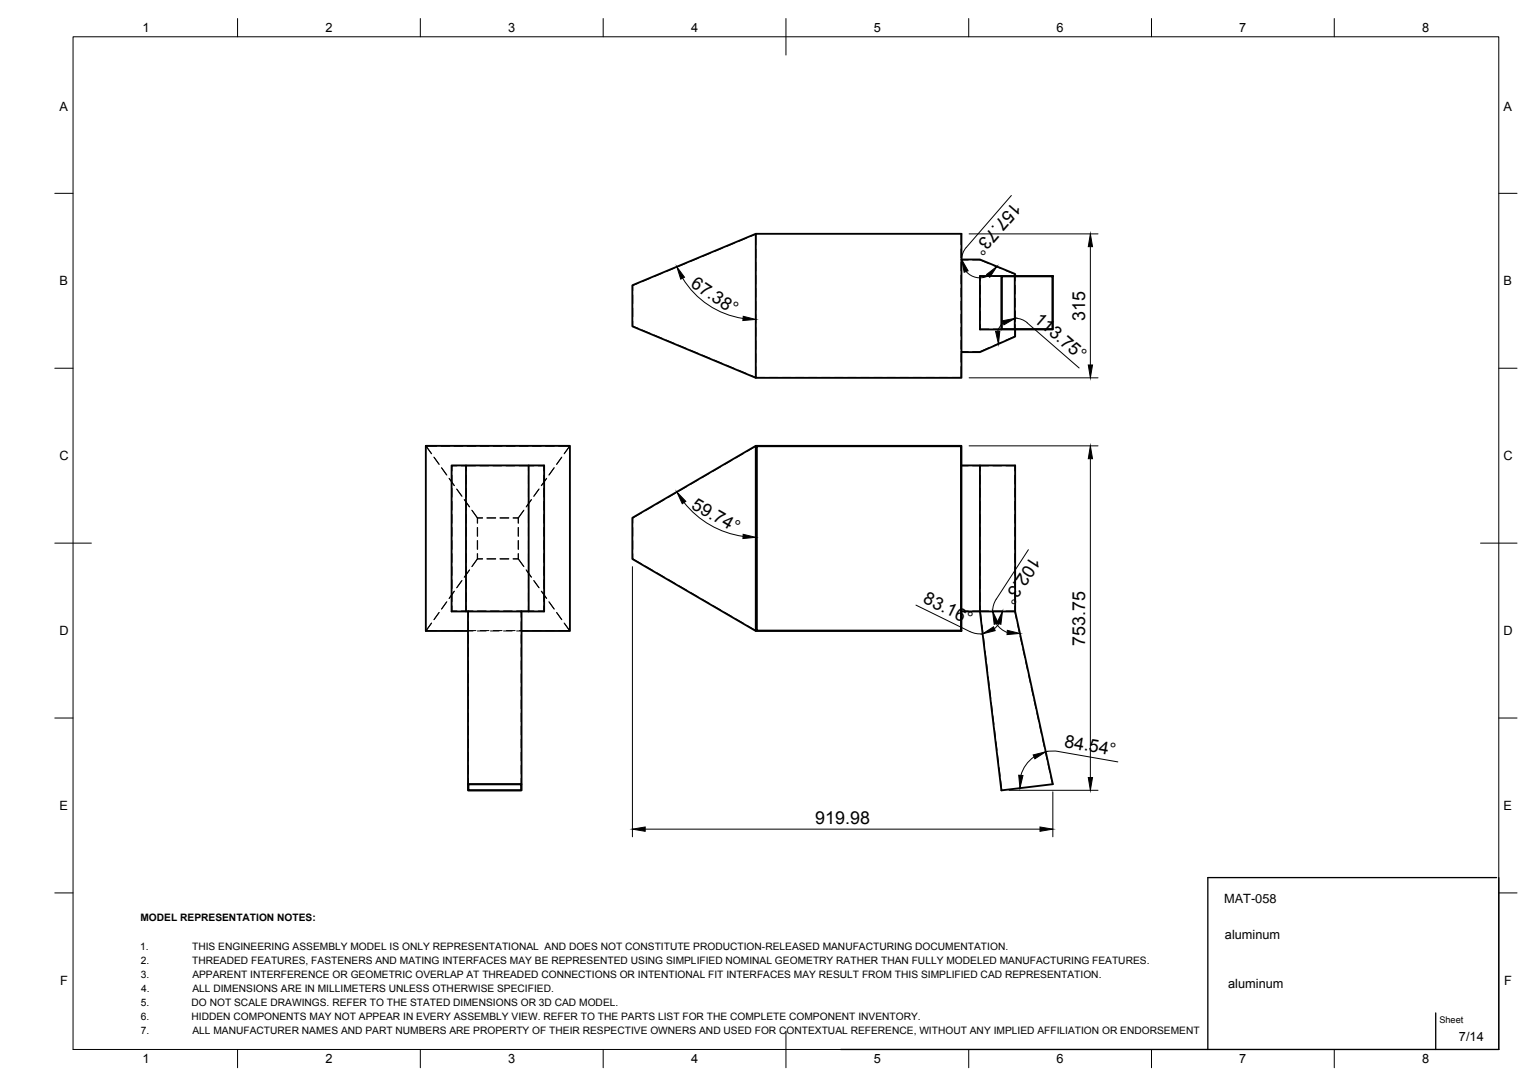
ISO-10303-21;
HEADER;
FILE_DESCRIPTION (('STEP AP214'),
    '1' );
FILE_NAME ('aluminum.step',
    '2026-10-21T17:54:40',
    ( '' ),
    ( '' ),
    'SwSTEP 2.0',
    'SolidWorks 2026',
    '' );
FILE_SCHEMA (( 'AUTOMOTIVE_DESIGN' ));
ENDSEC;

DATA;
#241=CARTESIAN_POINT ( 'NONE',  ( -208.1473046169136580, -154.8119894309599260, 472.8425600500171981 ) ) ;
#279=ORIENTED_EDGE ( 'NONE', *, *, #33326, .F. ) ;
#332=DIRECTION ( 'NONE',  ( 0.000000000000000000, -1.000000000000000000, 0.000000000000000000 ) ) ;
#357=VERTEX_POINT ( 'NONE', #3480 ) ;
#385=DIRECTION ( 'NONE',  ( 0.000000000000000000, -1.000000000000000000, 0.000000000000000000 ) ) ;
#451=CARTESIAN_POINT ( 'NONE',  ( -5.647304616913629616, 54.43801056904005975, 22.84256005001721945 ) ) ;
#457=CARTESIAN_POINT ( 'NONE',  ( 153.2026953830863647, 69.44873401059479079, -93.79675437945476801 ) ) ;
#484=DIRECTION ( 'NONE',  ( 0.1191452206184307472, 0.000000000000000000, -0.9928768384869219865 ) ) ;
#499=VECTOR ( 'NONE', #28091, 1000.000000000000000 ) ;
#615=DIRECTION ( 'NONE',  ( -0.000000000000000000, -1.000000000000000000, 0.000000000000000000 ) ) ;
#668=ORIENTED_EDGE ( 'NONE', *, *, #6729, .T. ) ;
#693=DIRECTION ( 'NONE',  ( 0.000000000000000000, -0.000000000000000000, 1.000000000000000000 ) ) ;
#702=ORIENTED_EDGE ( 'NONE', *, *, #9302, .T. ) ;
#814=CARTESIAN_POINT ( 'NONE',  ( -208.1473046169136580, -154.8119894309599260, 472.8425600500171981 ) ) ;
#959=ORIENTED_EDGE ( 'NONE', *, *, #6440, .T. ) ;
#975=CARTESIAN_POINT ( 'NONE',  ( 370.7621192902014968, 70.03596893647589638, -94.69675437945477370 ) ) ;
#987=DIRECTION ( 'NONE',  ( 1.000000000000000000, 0.000000000000000000, 0.000000000000000000 ) ) ;
#1016=VERTEX_POINT ( 'NONE', #25216 ) ;
#1060=EDGE_CURVE ( 'NONE', #41472, #40281, #17516, .T. ) ;
#1066=EDGE_CURVE ( 'NONE', #38528, #20059, #40122, .T. ) ;
#1071=ORIENTED_EDGE ( 'NONE', *, *, #6720, .F. ) ;
#1073=VECTOR ( 'NONE', #36151, 1000.000000000000114 ) ;
#1156=VECTOR ( 'NONE', #18949, 1000.000000000000000 ) ;
#1211=VERTEX_POINT ( 'NONE', #8004 ) ;
#1227=ORIENTED_EDGE ( 'NONE', *, *, #36593, .T. ) ;
#1314=VECTOR ( 'NONE', #13309, 1000.000000000000114 ) ;
#1326=ORIENTED_EDGE ( 'NONE', *, *, #18380, .F. ) ;
#1347=VECTOR ( 'NONE', #6757, 1000.000000000000114 ) ;
#1376=ADVANCED_FACE ( 'NONE', ( #40059 ), #40304, .F. ) ;
#1429=CARTESIAN_POINT ( 'NONE',  ( -556.8973046169135159, 54.43801056904003133, -64.63743994998280584 ) ) ;
#1492=LINE ( 'NONE', #20466, #38729 ) ;
#1712=DIRECTION ( 'NONE',  ( -1.000000000000000000, -0.000000000000000000, 0.000000000000000000 ) ) ;
#1716=CARTESIAN_POINT ( 'NONE',  ( 370.7621192902014968, 70.03596893647589638, -93.79675437945476801 ) ) ;
#1719=EDGE_CURVE ( 'NONE', #25392, #44652, #50206, .T. ) ;
#1752=ORIENTED_EDGE ( 'NONE', *, *, #22020, .F. ) ;
#1804=EDGE_CURVE ( 'NONE', #31856, #4890, #4338, .T. ) ;
#1839=FACE_OUTER_BOUND ( 'NONE', #12739, .T. ) ;
#1958=ORIENTED_EDGE ( 'NONE', *, *, #22698, .T. ) ;
#2000=CARTESIAN_POINT ( 'NONE',  ( -164.4973046169135955, -66.40178110878292728, -93.79675437945473959 ) ) ;
#2068=LINE ( 'NONE', #13349, #48206 ) ;
#2078=VECTOR ( 'NONE', #9444, 1000.000000000000227 ) ;
#2117=DIRECTION ( 'NONE',  ( 0.000000000000000000, -0.9253776417389547593, -0.3790464617558786942 ) ) ;
#2152=LINE ( 'NONE', #37326, #22207 ) ;
#2162=EDGE_LOOP ( 'NONE', ( #42165, #11431, #22910, #39612 ) ) ;
#2201=FACE_OUTER_BOUND ( 'NONE', #47299, .T. ) ;
#2211=ORIENTED_EDGE ( 'NONE', *, *, #2519, .F. ) ;
#2213=CARTESIAN_POINT ( 'NONE',  ( -5.647304616913629616, 160.1880105690400171, 472.8425600500173118 ) ) ;
#2225=ORIENTED_EDGE ( 'NONE', *, *, #29896, .T. ) ;
#2275=FACE_OUTER_BOUND ( 'NONE', #44624, .T. ) ;
#2284=ORIENTED_EDGE ( 'NONE', *, *, #38775, .F. ) ;
#2287=ADVANCED_FACE ( 'NONE', ( #1839 ), #41087, .T. ) ;
#2307=FACE_OUTER_BOUND ( 'NONE', #7610, .T. ) ;
#2377=PLANE ( 'NONE',  #19234 ) ;
#2481=CARTESIAN_POINT ( 'NONE',  ( 38.83576208387757589, 47.08801056904012228, 741.9425600500172777 ) ) ;
#2519=EDGE_CURVE ( 'NONE', #29402, #34186, #39530, .T. ) ;
#2583=CARTESIAN_POINT ( 'NONE',  ( -164.4973046169135955, 53.53801056904005407, -18.45589678844777382 ) ) ;
#2692=ADVANCED_FACE ( 'NONE', ( #36959 ), #36444, .T. ) ;
#2711=EDGE_LOOP ( 'NONE', ( #23565, #14957, #15394, #19348 ) ) ;
#2742=DIRECTION ( 'NONE',  ( -0.9770330068457271366, 0.000000000000000000, -0.2130880182788259247 ) ) ;
#2751=ORIENTED_EDGE ( 'NONE', *, *, #10925, .T. ) ;
#2770=AXIS2_PLACEMENT_3D ( 'NONE', #14804, #37669, #2742 ) ;
#2832=ORIENTED_EDGE ( 'NONE', *, *, #9784, .F. ) ;
#2859=ORIENTED_EDGE ( 'NONE', *, *, #15510, .T. ) ;
#2862=DIRECTION ( 'NONE',  ( 0.000000000000000000, 0.9152942571496521795, -0.4027858274925601445 ) ) ;
#2909=ORIENTED_EDGE ( 'NONE', *, *, #9784, .T. ) ;
#3005=CARTESIAN_POINT ( 'NONE',  ( 154.1026953830863420, -98.56198943095992604, -17.65743994998277699 ) ) ;
#3023=EDGE_LOOP ( 'NONE', ( #44750, #47253, #35868, #13821, #14713 ) ) ;
#3087=LINE ( 'NONE', #10042, #48814 ) ;
#3208=VECTOR ( 'NONE', #19916, 1000.000000000000000 ) ;
#3242=FACE_OUTER_BOUND ( 'NONE', #8976, .T. ) ;
#3351=DIRECTION ( 'NONE',  ( 0.000000000000000000, 0.000000000000000000, 1.000000000000000000 ) ) ;
#3374=VECTOR ( 'NONE', #29459, 1000.000000000000000 ) ;
#3480=CARTESIAN_POINT ( 'NONE',  ( -50.64730461691362962, -42.31198943095992604, 742.8425600500171413 ) ) ;
#3541=LINE ( 'NONE', #46871, #45418 ) ;
#3553=EDGE_CURVE ( 'NONE', #20088, #22621, #48242, .T. ) ;
#3577=AXIS2_PLACEMENT_3D ( 'NONE', #25346, #33059, #13534 ) ;
#3706=PLANE ( 'NONE',  #4301 ) ;
#3725=VERTEX_POINT ( 'NONE', #8741 ) ;
#3735=EDGE_CURVE ( 'NONE', #42730, #27480, #4375, .T. ) ;
#3758=ORIENTED_EDGE ( 'NONE', *, *, #8894, .F. ) ;
#3817=CARTESIAN_POINT ( 'NONE',  ( 39.35269538308637038, 47.68801056904006685, 742.8425600500171413 ) ) ;
#3834=ORIENTED_EDGE ( 'NONE', *, *, #4571, .F. ) ;
#3908=LINE ( 'NONE', #10652, #47749 ) ;
#3911=CARTESIAN_POINT ( 'NONE',  ( -164.4973046169135955, 53.53801056904001854, -93.79675437945476801 ) ) ;
#3928=ADVANCED_FACE ( 'NONE', ( #17684 ), #5622, .T. ) ;
#3938=ORIENTED_EDGE ( 'NONE', *, *, #33386, .F. ) ;
#4009=CARTESIAN_POINT ( 'NONE',  ( -164.4973046169135955, 70.03596893647589638, -93.79675437945476801 ) ) ;
#4016=CARTESIAN_POINT ( 'NONE',  ( -50.64730461691362962, -42.31198943095992604, 742.8425600500171413 ) ) ;
#4070=CARTESIAN_POINT ( 'NONE',  ( -556.8973046169135159, 54.43801056904003133, -64.63743994998280584 ) ) ;
#4096=ORIENTED_EDGE ( 'NONE', *, *, #42266, .F. ) ;
#4099=CARTESIAN_POINT ( 'NONE',  ( 154.1026953830863420, -67.00570555996102939, -94.69675437945474528 ) ) ;
#4135=VECTOR ( 'NONE', #44345, 1000.000000000000000 ) ;
#4150=LINE ( 'NONE', #814, #47619 ) ;
#4152=PLANE ( 'NONE',  #16321 ) ;
#4171=ORIENTED_EDGE ( 'NONE', *, *, #43549, .T. ) ;
#4211=FACE_OUTER_BOUND ( 'NONE', #5918, .T. ) ;
#4264=EDGE_CURVE ( 'NONE', #31874, #20963, #40978, .T. ) ;
#4301=AXIS2_PLACEMENT_3D ( 'NONE', #34514, #22695, #42690 ) ;
#4310=ORIENTED_EDGE ( 'NONE', *, *, #9209, .F. ) ;
#4325=DIRECTION ( 'NONE',  ( -1.000000000000000000, 0.000000000000000000, 0.000000000000000000 ) ) ;
#4338=LINE ( 'NONE', #16901, #24087 ) ;
#4351=ADVANCED_FACE ( 'NONE', ( #49381 ), #30436, .F. ) ;
#4375=LINE ( 'NONE', #35702, #16325 ) ;
#4413=CARTESIAN_POINT ( 'NONE',  ( -208.1473046169136580, 160.1880105690400171, 22.84256005001721945 ) ) ;
#4427=ORIENTED_EDGE ( 'NONE', *, *, #32748, .F. ) ;
#4434=ORIENTED_EDGE ( 'NONE', *, *, #15392, .T. ) ;
#4470=LINE ( 'NONE', #47025, #32763 ) ;
#4506=ORIENTED_EDGE ( 'NONE', *, *, #50675, .F. ) ;
#4518=LINE ( 'NONE', #47068, #26246 ) ;
#4571=EDGE_CURVE ( 'NONE', #27616, #3725, #12944, .T. ) ;
#4605=VECTOR ( 'NONE', #22848, 1000.000000000000000 ) ;
#4617=EDGE_LOOP ( 'NONE', ( #15516, #44597, #12349, #35678 ) ) ;
#4639=EDGE_CURVE ( 'NONE', #46409, #16952, #10550, .T. ) ;
#4661=CARTESIAN_POINT ( 'NONE',  ( 196.8526953830863135, -154.8119894309599260, 472.8425600500171981 ) ) ;
#4676=DIRECTION ( 'NONE',  ( 0.000000000000000000, -0.3846153846153845812, -0.9230769230769231282 ) ) ;
#4704=EDGE_CURVE ( 'NONE', #36023, #25767, #19001, .T. ) ;
#4730=LINE ( 'NONE', #31435, #48310 ) ;
#4735=VERTEX_POINT ( 'NONE', #22856 ) ;
#4773=LINE ( 'NONE', #12731, #46270 ) ;
#4832=EDGE_CURVE ( 'NONE', #357, #47536, #47438, .T. ) ;
#4867=VERTEX_POINT ( 'NONE', #43124 ) ;
#4873=DIRECTION ( 'NONE',  ( 1.000000000000000000, 0.000000000000000000, 0.000000000000000000 ) ) ;
#4878=AXIS2_PLACEMENT_3D ( 'NONE', #40789, #12566, #28740 ) ;
#4890=VERTEX_POINT ( 'NONE', #8239 ) ;
#4959=CARTESIAN_POINT ( 'NONE',  ( -164.4973046169135955, 69.44873401059479079, -93.79675437945476801 ) ) ;
#5068=DIRECTION ( 'NONE',  ( 0.000000000000000000, -0.9253776417389547593, -0.3790464617558786942 ) ) ;
#5165=EDGE_CURVE ( 'NONE', #30282, #4735, #15614, .T. ) ;
#5212=DIRECTION ( 'NONE',  ( 0.000000000000000000, -1.000000000000000000, -0.000000000000000000 ) ) ;
#5272=AXIS2_PLACEMENT_3D ( 'NONE', #1716, #29409, #36381 ) ;
#5316=ORIENTED_EDGE ( 'NONE', *, *, #3735, .F. ) ;
#5368=ORIENTED_EDGE ( 'NONE', *, *, #46578, .T. ) ;
#5378=PLANE ( 'NONE',  #4878 ) ;
#5502=ORIENTED_EDGE ( 'NONE', *, *, #31003, .F. ) ;
#5540=AXIS2_PLACEMENT_3D ( 'NONE', #24472, #5212, #47523 ) ;
#5555=FACE_OUTER_BOUND ( 'NONE', #35797, .T. ) ;
#5588=FACE_OUTER_BOUND ( 'NONE', #2162, .T. ) ;
#5622=PLANE ( 'NONE',  #46600 ) ;
#5653=DIRECTION ( 'NONE',  ( 0.5038710255240859137, 0.000000000000000000, -0.8637789008984335659 ) ) ;
#5658=VECTOR ( 'NONE', #45006, 1000.000000000000114 ) ;
#5681=AXIS2_PLACEMENT_3D ( 'NONE', #34207, #37561, #30098 ) ;
#5701=PLANE ( 'NONE',  #34925 ) ;
#5715=CARTESIAN_POINT ( 'NONE',  ( -207.2473046169136808, -153.9383703589661252, 472.5992458228021746 ) ) ;
#5732=CARTESIAN_POINT ( 'NONE',  ( 370.7621192902014968, -66.40178110878291307, -93.79675437945473959 ) ) ;
#5757=ORIENTED_EDGE ( 'NONE', *, *, #34999, .T. ) ;
#5892=EDGE_LOOP ( 'NONE', ( #32196, #5502, #38784, #26023 ) ) ;
#5918=EDGE_LOOP ( 'NONE', ( #14911, #33689, #33782, #18625 ) ) ;
#5973=CARTESIAN_POINT ( 'NONE',  ( -164.4973046169135955, -61.66198943095990614, -93.79675437945473959 ) ) ;
#6037=DIRECTION ( 'NONE',  ( -0.9928768384869220975, 0.000000000000000000, -0.1191452206184307611 ) ) ;
#6163=ORIENTED_EDGE ( 'NONE', *, *, #39420, .F. ) ;
#6228=VECTOR ( 'NONE', #30490, 1000.000000000000000 ) ;
#6308=AXIS2_PLACEMENT_3D ( 'NONE', #19441, #11251, #26887 ) ;
#6387=ORIENTED_EDGE ( 'NONE', *, *, #14417, .F. ) ;
#6440=EDGE_CURVE ( 'NONE', #13303, #25392, #15576, .T. ) ;
#6451=CARTESIAN_POINT ( 'NONE',  ( 195.9526953830863079, -154.8119894309599260, 472.8425600500171981 ) ) ;
#6643=CARTESIAN_POINT ( 'NONE',  ( -50.64730461691362962, 47.68801056904006685, 742.8425600500171413 ) ) ;
#6720=EDGE_CURVE ( 'NONE', #26345, #33351, #34012, .T. ) ;
#6726=ADVANCED_FACE ( 'NONE', ( #2201, #48848 ), #49598, .T. ) ;
#6729=EDGE_CURVE ( 'NONE', #4735, #33351, #37872, .T. ) ;
#6757=DIRECTION ( 'NONE',  ( 0.000000000000000000, 0.3790464617558786942, -0.9253776417389547593 ) ) ;
#6766=DIRECTION ( 'NONE',  ( 0.000000000000000000, 0.4027858274925601445, 0.9152942571496521795 ) ) ;
#6768=ORIENTED_EDGE ( 'NONE', *, *, #46179, .F. ) ;
#6777=ORIENTED_EDGE ( 'NONE', *, *, #27524, .F. ) ;
#6972=ORIENTED_EDGE ( 'NONE', *, *, #41993, .T. ) ;
#6980=AXIS2_PLACEMENT_3D ( 'NONE', #13034, #17149, #44560 ) ;
#6996=LINE ( 'NONE', #15633, #34336 ) ;
#7016=CARTESIAN_POINT ( 'NONE',  ( -208.1473046169136580, -154.8119894309599260, 22.84256005001721945 ) ) ;
#7047=CARTESIAN_POINT ( 'NONE',  ( 39.35269538308637038, 47.68801056904006685, 742.8425600500171413 ) ) ;
#7067=VECTOR ( 'NONE', #31546, 999.9999999999998863 ) ;
#7103=LINE ( 'NONE', #4009, #35899 ) ;
#7136=DIRECTION ( 'NONE',  ( 0.000000000000000000, 1.000000000000000000, 0.000000000000000000 ) ) ;
#7199=DIRECTION ( 'NONE',  ( 1.000000000000000000, -0.000000000000000000, 0.000000000000000000 ) ) ;
#7200=VERTEX_POINT ( 'NONE', #19803 ) ;
#7296=CARTESIAN_POINT ( 'NONE',  ( 38.83576208387763273, -41.71198943095993172, 741.9425600500172777 ) ) ;
#7407=EDGE_CURVE ( 'NONE', #12974, #48624, #12867, .T. ) ;
#7419=ORIENTED_EDGE ( 'NONE', *, *, #33361, .F. ) ;
#7497=CARTESIAN_POINT ( 'NONE',  ( -556.8973046169135159, -62.56198943095993315, -64.63743994998280584 ) ) ;
#7575=FACE_OUTER_BOUND ( 'NONE', #40709, .T. ) ;
#7610=EDGE_LOOP ( 'NONE', ( #10377, #45891, #20577, #22178 ) ) ;
#7656=ORIENTED_EDGE ( 'NONE', *, *, #1804, .F. ) ;
#7677=CARTESIAN_POINT ( 'NONE',  ( 370.7621192902014968, -61.66198943095990614, -93.79675437945473959 ) ) ;
#7727=ORIENTED_EDGE ( 'NONE', *, *, #31034, .F. ) ;
#7759=ORIENTED_EDGE ( 'NONE', *, *, #34938, .F. ) ;
#7761=DIRECTION ( 'NONE',  ( 0.000000000000000000, -0.9230769230769231282, 0.3846153846153845812 ) ) ;
#7783=DIRECTION ( 'NONE',  ( 0.000000000000000000, 0.000000000000000000, -1.000000000000000000 ) ) ;
#7797=PLANE ( 'NONE',  #11121 ) ;
#7813=DIRECTION ( 'NONE',  ( 0.000000000000000000, 0.000000000000000000, 1.000000000000000000 ) ) ;
#7846=( GEOMETRIC_REPRESENTATION_CONTEXT ( 3 ) GLOBAL_UNCERTAINTY_ASSIGNED_CONTEXT ( ( #27104 ) ) GLOBAL_UNIT_ASSIGNED_CONTEXT ( ( #23127, #47956, #47455 ) ) REPRESENTATION_CONTEXT ( 'NONE', 'WORKASPACE' ) );
#7878=CARTESIAN_POINT ( 'NONE',  ( 196.8526953830863420, -154.8119894309599260, 472.8425600500170844 ) ) ;
#7879=VECTOR ( 'NONE', #40972, 1000.000000000000000 ) ;
#7909=VECTOR ( 'NONE', #41910, 1000.000000000000000 ) ;
#8004=CARTESIAN_POINT ( 'NONE',  ( -207.2473046169136808, -154.8119894309599260, 23.74256005001722158 ) ) ;
#8048=DIRECTION ( 'NONE',  ( 0.5038710255240862468, 0.000000000000000000, 0.8637789008984334549 ) ) ;
#8050=FACE_OUTER_BOUND ( 'NONE', #9334, .T. ) ;
#8121=VECTOR ( 'NONE', #23458, 1000.000000000000000 ) ;
#8149=PLANE ( 'NONE',  #11807 ) ;
#8154=DIRECTION ( 'NONE',  ( 0.4740998230350172427, -0.3386427307392981811, -0.8127425537743158124 ) ) ;
#8166=DIRECTION ( 'NONE',  ( 0.000000000000000000, -1.000000000000000000, 0.000000000000000000 ) ) ;
#8168=ORIENTED_EDGE ( 'NONE', *, *, #31034, .T. ) ;
#8177=DIRECTION ( 'NONE',  ( -1.000000000000000000, 0.000000000000000000, 0.000000000000000000 ) ) ;
#8179=PLANE ( 'NONE',  #37093 ) ;
#8217=ORIENTED_EDGE ( 'NONE', *, *, #36565, .F. ) ;
#8239=CARTESIAN_POINT ( 'NONE',  ( 154.1026953830863420, 103.9380105690400597, 22.84256005001721945 ) ) ;
#8319=CARTESIAN_POINT ( 'NONE',  ( -165.2900739183569954, 53.53801056904005407, -18.55102910462098365 ) ) ;
#8510=AXIS2_PLACEMENT_3D ( 'NONE', #18220, #7199, #38007 ) ;
#8516=FACE_OUTER_BOUND ( 'NONE', #34229, .T. ) ;
#8566=DIRECTION ( 'NONE',  ( -0.000000000000000000, -0.000000000000000000, 1.000000000000000000 ) ) ;
#8605=ORIENTED_EDGE ( 'NONE', *, *, #19335, .F. ) ;
#8741=CARTESIAN_POINT ( 'NONE',  ( -165.4943081650521037, -61.66198943095990614, -93.79675437945473959 ) ) ;
#8749=FACE_OUTER_BOUND ( 'NONE', #17973, .T. ) ;
#8894=EDGE_CURVE ( 'NONE', #17600, #41530, #24626, .T. ) ;
#8916=CARTESIAN_POINT ( 'NONE',  ( 38.83576208387761142, 2.688010569040066411, 741.9425600500172777 ) ) ;
#8953=EDGE_CURVE ( 'NONE', #46082, #3725, #25376, .T. ) ;
#8976=EDGE_LOOP ( 'NONE', ( #44232, #3834, #6777, #10085 ) ) ;
#9036=VECTOR ( 'NONE', #484, 1000.000000000000114 ) ;
#9112=AXIS2_PLACEMENT_3D ( 'NONE', #41445, #6037, #37378 ) ;
#9190=VECTOR ( 'NONE', #44606, 1000.000000000000000 ) ;
#9209=EDGE_CURVE ( 'NONE', #15492, #38770, #29639, .T. ) ;
#9216=EDGE_CURVE ( 'NONE', #4735, #20088, #10137, .T. ) ;
#9302=EDGE_CURVE ( 'NONE', #14628, #1211, #26754, .T. ) ;
#9334=EDGE_LOOP ( 'NONE', ( #18121, #13690, #6387, #16671 ) ) ;
#9439=CARTESIAN_POINT ( 'NONE',  ( -5.647304616913629616, 159.2880105690400399, 23.74256005001722158 ) ) ;
#9444=DIRECTION ( 'NONE',  ( -0.4740998230350175202, 0.3386427307392980146, -0.8127425537743157014 ) ) ;
#9449=DIRECTION ( 'NONE',  ( 1.000000000000000000, 0.000000000000000000, 0.000000000000000000 ) ) ;
#9475=DIRECTION ( 'NONE',  ( 0.000000000000000000, -0.3846153846153844702, 0.9230769230769231282 ) ) ;
#9516=EDGE_CURVE ( 'NONE', #32226, #1016, #48227, .T. ) ;
#9520=EDGE_CURVE ( 'NONE', #27480, #28855, #13116, .T. ) ;
#9532=ORIENTED_EDGE ( 'NONE', *, *, #1066, .F. ) ;
#9600=EDGE_CURVE ( 'NONE', #25574, #4867, #25688, .T. ) ;
#9643=ORIENTED_EDGE ( 'NONE', *, *, #4832, .F. ) ;
#9657=VERTEX_POINT ( 'NONE', #12240 ) ;
#9658=LINE ( 'NONE', #34277, #11469 ) ;
#9686=PLANE ( 'NONE',  #32506 ) ;
#9784=EDGE_CURVE ( 'NONE', #21642, #20088, #28904, .T. ) ;
#9799=EDGE_CURVE ( 'NONE', #42832, #20659, #24809, .T. ) ;
#9967=DIRECTION ( 'NONE',  ( 0.000000000000000000, -1.000000000000000000, 0.000000000000000000 ) ) ;
#10013=PLANE ( 'NONE',  #40935 ) ;
#10019=EDGE_CURVE ( 'NONE', #48624, #30357, #16041, .T. ) ;
#10042=CARTESIAN_POINT ( 'NONE',  ( 196.8526953830862567, 2.688010569040066411, 472.8425600500171981 ) ) ;
#10072=DIRECTION ( 'NONE',  ( 0.8637789008984335659, -0.000000000000000000, 0.5038710255240859137 ) ) ;
#10078=CARTESIAN_POINT ( 'NONE',  ( 370.7621192902014968, 103.1142457376053727, -17.29493270523947501 ) ) ;
#10079=VECTOR ( 'NONE', #9449, 1000.000000000000000 ) ;
#10085=ORIENTED_EDGE ( 'NONE', *, *, #14919, .T. ) ;
#10137=LINE ( 'NONE', #10640, #5658 ) ;
#10241=DIRECTION ( 'NONE',  ( 0.000000000000000000, 0.9230769230769231282, 0.3846153846153844702 ) ) ;
#10271=CARTESIAN_POINT ( 'NONE',  ( 341.2957005644334458, 2.688010569040066411, 225.2259797391361644 ) ) ;
#10274=EDGE_LOOP ( 'NONE', ( #45472, #29853, #38354, #1958 ) ) ;
#10283=CARTESIAN_POINT ( 'NONE',  ( 154.1026953830863420, -98.56198943095992604, 22.84256005001721945 ) ) ;
#10287=DIRECTION ( 'NONE',  ( -0.000000000000000000, -0.000000000000000000, -1.000000000000000000 ) ) ;
#10334=CARTESIAN_POINT ( 'NONE',  ( -208.1473046169136580, 159.2880105690400399, 472.8425600500171981 ) ) ;
#10343=VECTOR ( 'NONE', #20955, 1000.000000000000000 ) ;
#10370=ORIENTED_EDGE ( 'NONE', *, *, #22698, .F. ) ;
#10377=ORIENTED_EDGE ( 'NONE', *, *, #33550, .T. ) ;
#10415=ORIENTED_EDGE ( 'NONE', *, *, #30569, .F. ) ;
#10441=ORIENTED_EDGE ( 'NONE', *, *, #38193, .F. ) ;
#10514=VERTEX_POINT ( 'NONE', #12619 ) ;
#10550=LINE ( 'NONE', #6451, #13168 ) ;
#10572=PRODUCT_DEFINITION_SHAPE ( 'NONE', 'NONE',  #26547 ) ;
#10590=VECTOR ( 'NONE', #15446, 1000.000000000000114 ) ;
#10640=CARTESIAN_POINT ( 'NONE',  ( -543.3973046169135159, 54.43801056904003133, -177.1374399499827916 ) ) ;
#10652=CARTESIAN_POINT ( 'NONE',  ( 39.35269538308637038, -42.31198943095992604, 742.8425600500171413 ) ) ;
#10663=CARTESIAN_POINT ( 'NONE',  ( -543.3973046169135159, -62.56198943095993315, -177.1374399499827916 ) ) ;
#10687=CARTESIAN_POINT ( 'NONE',  ( 153.2026953830863647, 103.0380105690400683, 23.74256005001722158 ) ) ;
#10726=EDGE_CURVE ( 'NONE', #25574, #42832, #3087, .T. ) ;
#10747=DIRECTION ( 'NONE',  ( 0.000000000000000000, -0.000000000000000000, 1.000000000000000000 ) ) ;
#10757=CARTESIAN_POINT ( 'NONE',  ( 153.2026953830863647, 70.03596893647589638, -93.79675437945476801 ) ) ;
#10831=FACE_OUTER_BOUND ( 'NONE', #17866, .T. ) ;
#10925=EDGE_CURVE ( 'NONE', #14108, #41530, #43605, .T. ) ;
#10942=DIRECTION ( 'NONE',  ( 0.000000000000000000, -1.000000000000000000, 1.822804496942680012E-16 ) ) ;
#11100=AXIS2_PLACEMENT_3D ( 'NONE', #241, #43314, #23577 ) ;
#11121=AXIS2_PLACEMENT_3D ( 'NONE', #30377, #27025, #6766 ) ;
#11175=ADVANCED_FACE ( 'NONE', ( #30750 ), #46358, .F. ) ;
#11246=ORIENTED_EDGE ( 'NONE', *, *, #1060, .T. ) ;
#11251=DIRECTION ( 'NONE',  ( 0.000000000000000000, 0.9230769230769231282, 0.3846153846153844702 ) ) ;
#11268=VECTOR ( 'NONE', #32064, 1000.000000000000000 ) ;
#11272=PLANE ( 'NONE',  #11100 ) ;
#11320=CARTESIAN_POINT ( 'NONE',  ( 153.2026953830863647, -97.72914955339486198, -17.31629813440246579 ) ) ;
#11328=ORIENTED_EDGE ( 'NONE', *, *, #19813, .T. ) ;
#11393=DIRECTION ( 'NONE',  ( 0.000000000000000000, 0.000000000000000000, -1.000000000000000000 ) ) ;
#11397=VERTEX_POINT ( 'NONE', #38592 ) ;
#11431=ORIENTED_EDGE ( 'NONE', *, *, #42525, .F. ) ;
#11469=VECTOR ( 'NONE', #41203, 999.9999999999998863 ) ;
#11632=ORIENTED_EDGE ( 'NONE', *, *, #32563, .F. ) ;
#11681=LINE ( 'NONE', #15027, #31653 ) ;
#11733=DIRECTION ( 'NONE',  ( 0.000000000000000000, 1.000000000000000000, 0.000000000000000000 ) ) ;
#11807=AXIS2_PLACEMENT_3D ( 'NONE', #451, #16094, #693 ) ;
#11836=ORIENTED_EDGE ( 'NONE', *, *, #29635, .T. ) ;
#11911=CARTESIAN_POINT ( 'NONE',  ( -165.3973046169136012, -98.56198943095992604, -17.65743994998277699 ) ) ;
#11924=CARTESIAN_POINT ( 'NONE',  ( 154.1026953830863420, 70.03596893647589638, -94.69675437945477370 ) ) ;
#12017=VECTOR ( 'NONE', #47379, 1000.000000000000000 ) ;
#12064=EDGE_LOOP ( 'NONE', ( #38247, #45848, #34785, #1752 ) ) ;
#12089=ADVANCED_FACE ( 'NONE', ( #32086 ), #5378, .T. ) ;
#12130=DIRECTION ( 'NONE',  ( -1.000000000000000000, 0.000000000000000000, -0.000000000000000000 ) ) ;
#12202=EDGE_LOOP ( 'NONE', ( #41677, #13801, #35310, #39306 ) ) ;
#12240=CARTESIAN_POINT ( 'NONE',  ( -556.7900739183570522, 53.53801056904005407, -65.53102910462104091 ) ) ;
#12305=CARTESIAN_POINT ( 'NONE',  ( -165.3973046169136012, 70.03596893647589638, -94.69675437945477370 ) ) ;
#12324=CARTESIAN_POINT ( 'NONE',  ( -50.64730461691362962, -42.31198943095992604, 742.8425600500171413 ) ) ;
#12345=AXIS2_PLACEMENT_3D ( 'NONE', #46084, #7136, #19167 ) ;
#12349=ORIENTED_EDGE ( 'NONE', *, *, #9216, .T. ) ;
#12406=CARTESIAN_POINT ( 'NONE',  ( 370.7621192902014968, 53.53801056904005407, -93.79675437945476801 ) ) ;
#12421=DIRECTION ( 'NONE',  ( 0.000000000000000000, -1.000000000000000000, 0.000000000000000000 ) ) ;
#12440=VERTEX_POINT ( 'NONE', #22795 ) ;
#12483=FACE_OUTER_BOUND ( 'NONE', #28221, .T. ) ;
#12522=LINE ( 'NONE', #17386, #29125 ) ;
#12557=DIRECTION ( 'NONE',  ( -1.000000000000000000, -0.000000000000000000, -0.000000000000000000 ) ) ;
#12566=DIRECTION ( 'NONE',  ( -1.000000000000000000, 0.000000000000000000, 0.000000000000000000 ) ) ;
#12619=CARTESIAN_POINT ( 'NONE',  ( 153.2026953830863647, 103.0380105690400683, -17.46817021067766973 ) ) ;
#12632=PLANE ( 'NONE',  #29185 ) ;
#12680=ORIENTED_EDGE ( 'NONE', *, *, #32509, .T. ) ;
#12706=( GEOMETRIC_REPRESENTATION_CONTEXT ( 3 ) GLOBAL_UNCERTAINTY_ASSIGNED_CONTEXT ( ( #46464 ) ) GLOBAL_UNIT_ASSIGNED_CONTEXT ( ( #48263, #45433, #26471 ) ) REPRESENTATION_CONTEXT ( 'NONE', 'WORKASPACE' ) );
#12726=VECTOR ( 'NONE', #32276, 1000.000000000000227 ) ;
#12729=EDGE_CURVE ( 'NONE', #1016, #46409, #46803, .T. ) ;
#12731=CARTESIAN_POINT ( 'NONE',  ( -164.4973046169135955, -98.56198943095992604, 23.74256005001722158 ) ) ;
#12739=EDGE_LOOP ( 'NONE', ( #38201, #21263, #26940, #38391 ) ) ;
#12837=VECTOR ( 'NONE', #16614, 1000.000000000000000 ) ;
#12845=CARTESIAN_POINT ( 'NONE',  ( -165.2900739183569954, 54.43801056904003133, -18.55102910462098365 ) ) ;
#12867=LINE ( 'NONE', #43648, #3374 ) ;
#12885=LINE ( 'NONE', #32399, #16951 ) ;
#12896=CARTESIAN_POINT ( 'NONE',  ( -208.1473046169136580, 2.688010569040066411, 472.8425600500171981 ) ) ;
#12943=ADVANCED_FACE ( 'NONE', ( #2307 ), #10013, .T. ) ;
#12944=LINE ( 'NONE', #32477, #20528 ) ;
#12974=VERTEX_POINT ( 'NONE', #37247 ) ;
#13018=VECTOR ( 'NONE', #26188, 1000.000000000000000 ) ;
#13030=DIRECTION ( 'NONE',  ( -1.000000000000000000, 0.000000000000000000, 0.000000000000000000 ) ) ;
#13034=CARTESIAN_POINT ( 'NONE',  ( 154.1026953830863420, -97.66198943095992036, -17.65743994998277699 ) ) ;
#13116=LINE ( 'NONE', #28777, #13018 ) ;
#13119=PLANE ( 'NONE',  #13393 ) ;
#13121=DIRECTION ( 'NONE',  ( 0.9770330068457271366, -0.000000000000000000, 0.2130880182788259247 ) ) ;
#13135=DIRECTION ( 'NONE',  ( -0.000000000000000000, -0.000000000000000000, 1.000000000000000000 ) ) ;
#13168=VECTOR ( 'NONE', #26215, 1000.000000000000000 ) ;
#13193=VERTEX_POINT ( 'NONE', #24599 ) ;
#13205=ORIENTED_EDGE ( 'NONE', *, *, #32827, .T. ) ;
#13270=CARTESIAN_POINT ( 'NONE',  ( -50.13037131770486354, 2.688010569040066411, 741.9425600500171640 ) ) ;
#13303=VERTEX_POINT ( 'NONE', #2000 ) ;
#13309=DIRECTION ( 'NONE',  ( 0.9770330068457271366, 0.000000000000000000, 0.2130880182788258970 ) ) ;
#13334=ORIENTED_EDGE ( 'NONE', *, *, #3735, .T. ) ;
#13349=CARTESIAN_POINT ( 'NONE',  ( -556.7900739183570522, 54.43801056904003133, -65.53102910462104091 ) ) ;
#13393=AXIS2_PLACEMENT_3D ( 'NONE', #45403, #37016, #33156 ) ;
#13406=DIRECTION ( 'NONE',  ( 0.000000000000000000, -0.000000000000000000, -1.000000000000000000 ) ) ;
#13534=DIRECTION ( 'NONE',  ( -1.000000000000000000, 0.000000000000000000, -0.000000000000000000 ) ) ;
#13538=PLANE ( 'NONE',  #6980 ) ;
#13563=EDGE_CURVE ( 'NONE', #4867, #29402, #20174, .T. ) ;
#13630=DIRECTION ( 'NONE',  ( 0.000000000000000000, 0.000000000000000000, -1.000000000000000000 ) ) ;
#13690=ORIENTED_EDGE ( 'NONE', *, *, #1060, .F. ) ;
#13762=DIRECTION ( 'NONE',  ( 0.000000000000000000, 1.000000000000000000, 0.000000000000000000 ) ) ;
#13780=PLANE ( 'NONE',  #3577 ) ;
#13792=CARTESIAN_POINT ( 'NONE',  ( 39.35269538308637038, -42.31198943095992604, 742.8425600500171413 ) ) ;
#13801=ORIENTED_EDGE ( 'NONE', *, *, #9600, .F. ) ;
#13821=ORIENTED_EDGE ( 'NONE', *, *, #16934, .F. ) ;
#14034=FACE_OUTER_BOUND ( 'NONE', #34092, .T. ) ;
#14108=VERTEX_POINT ( 'NONE', #4099 ) ;
#14153=LINE ( 'NONE', #25217, #14583 ) ;
#14371=VECTOR ( 'NONE', #13121, 1000.000000000000114 ) ;
#14417=EDGE_CURVE ( 'NONE', #23001, #41472, #42267, .T. ) ;
#14446=ORIENTED_EDGE ( 'NONE', *, *, #12729, .F. ) ;
#14455=AXIS2_PLACEMENT_3D ( 'NONE', #14910, #38536, #3351 ) ;
#14583=VECTOR ( 'NONE', #17770, 1000.000000000000000 ) ;
#14591=ORIENTED_EDGE ( 'NONE', *, *, #17350, .T. ) ;
#14598=DIRECTION ( 'NONE',  ( 0.000000000000000000, 1.000000000000000000, 0.000000000000000000 ) ) ;
#14628=VERTEX_POINT ( 'NONE', #32003 ) ;
#14641=ORIENTED_EDGE ( 'NONE', *, *, #6720, .T. ) ;
#14677=PRODUCT ( 'aluminum', 'aluminum', '', ( #16450 ) ) ;
#14681=PLANE ( 'NONE',  #27228 ) ;
#14705=ADVANCED_FACE ( 'NONE', ( #44514 ), #21437, .T. ) ;
#14713=ORIENTED_EDGE ( 'NONE', *, *, #50581, .F. ) ;
#14745=DIRECTION ( 'NONE',  ( -1.000000000000000000, 0.000000000000000000, 0.000000000000000000 ) ) ;
#14804=CARTESIAN_POINT ( 'NONE',  ( -543.5890838333644979, 54.43801056904003133, -176.2581102438216192 ) ) ;
#14805=ORIENTED_EDGE ( 'NONE', *, *, #9520, .F. ) ;
#14837=CARTESIAN_POINT ( 'NONE',  ( -208.1473046169136580, 160.1880105690400171, 472.8425600500171981 ) ) ;
#14880=ORIENTED_EDGE ( 'NONE', *, *, #9799, .F. ) ;
#14910=CARTESIAN_POINT ( 'NONE',  ( 153.2026953830863647, -98.56198943095992604, -17.65743994998277699 ) ) ;
#14911=ORIENTED_EDGE ( 'NONE', *, *, #10019, .F. ) ;
#14919=EDGE_CURVE ( 'NONE', #13193, #46082, #4730, .T. ) ;
#14957=ORIENTED_EDGE ( 'NONE', *, *, #40873, .T. ) ;
#14977=EDGE_LOOP ( 'NONE', ( #36134, #24812, #14805, #5316, #7727, #40850, #31124, #30943, #31752, #10415 ) ) ;
#14981=VECTOR ( 'NONE', #21295, 1000.000000000000000 ) ;
#15027=CARTESIAN_POINT ( 'NONE',  ( -165.3973046169136012, -62.56198943095993315, -17.65743994998275213 ) ) ;
#15038=CARTESIAN_POINT ( 'NONE',  ( -208.1473046169136580, -154.8119894309599260, 472.8425600500171981 ) ) ;
#15084=CARTESIAN_POINT ( 'NONE',  ( 153.2026953830863647, -97.66198943095992036, -17.48025818148969890 ) ) ;
#15111=PLANE ( 'NONE',  #41066 ) ;
#15132=VERTEX_POINT ( 'NONE', #38827 ) ;
#15195=FACE_OUTER_BOUND ( 'NONE', #22326, .T. ) ;
#15268=FACE_OUTER_BOUND ( 'NONE', #32284, .T. ) ;
#15273=LINE ( 'NONE', #34260, #20484 ) ;
#15370=DIRECTION ( 'NONE',  ( -1.000000000000000000, 0.000000000000000000, 0.000000000000000000 ) ) ;
#15392=EDGE_CURVE ( 'NONE', #22621, #15132, #30478, .T. ) ;
#15394=ORIENTED_EDGE ( 'NONE', *, *, #19352, .T. ) ;
#15397=DIRECTION ( 'NONE',  ( 0.000000000000000000, 1.000000000000000000, -1.822804496942679766E-16 ) ) ;
#15434=DIRECTION ( 'NONE',  ( 0.000000000000000000, -1.000000000000000000, 0.000000000000000000 ) ) ;
#15446=DIRECTION ( 'NONE',  ( 0.000000000000000000, -0.4027858274925600890, -0.9152942571496521795 ) ) ;
#15492=VERTEX_POINT ( 'NONE', #35373 ) ;
#15502=ADVANCED_FACE ( 'NONE', ( #31004 ), #34858, .F. ) ;
#15507=VECTOR ( 'NONE', #29263, 1000.000000000000000 ) ;
#15510=EDGE_CURVE ( 'NONE', #31874, #15492, #19693, .T. ) ;
#15516=ORIENTED_EDGE ( 'NONE', *, *, #27935, .F. ) ;
#15550=VERTEX_POINT ( 'NONE', #457 ) ;
#15576=LINE ( 'NONE', #46831, #37804 ) ;
#15602=CARTESIAN_POINT ( 'NONE',  ( -208.1473046169136296, -154.8119894309598976, 472.8425600500173118 ) ) ;
#15612=VECTOR ( 'NONE', #9967, 1000.000000000000000 ) ;
#15614=LINE ( 'NONE', #4070, #9036 ) ;
#15633=CARTESIAN_POINT ( 'NONE',  ( -165.3973046169136012, -98.56198943095992604, 22.84256005001721945 ) ) ;
#15663=DIRECTION ( 'NONE',  ( 0.000000000000000000, -1.000000000000000000, 1.822804496942680012E-16 ) ) ;
#15696=DIRECTION ( 'NONE',  ( 0.000000000000000000, -0.3846153846153845812, -0.9230769230769231282 ) ) ;
#15697=ORIENTED_EDGE ( 'NONE', *, *, #45308, .F. ) ;
#15758=VECTOR ( 'NONE', #17300, 1000.000000000000000 ) ;
#15807=ORIENTED_EDGE ( 'NONE', *, *, #9302, .F. ) ;
#15812=CARTESIAN_POINT ( 'NONE',  ( 195.9526953830863079, -154.8119894309599260, 23.74256005001722158 ) ) ;
#15991=ORIENTED_EDGE ( 'NONE', *, *, #19352, .F. ) ;
#15998=ORIENTED_EDGE ( 'NONE', *, *, #9516, .T. ) ;
#16000=VECTOR ( 'NONE', #33063, 1000.000000000000000 ) ;
#16041=LINE ( 'NONE', #31953, #499 ) ;
#16075=LINE ( 'NONE', #4016, #25859 ) ;
#16091=CARTESIAN_POINT ( 'NONE',  ( -5.647304616913629616, 53.53801056904005407, 22.84256005001721945 ) ) ;
#16094=DIRECTION ( 'NONE',  ( 0.000000000000000000, 1.000000000000000000, 0.000000000000000000 ) ) ;
#16236=ORIENTED_EDGE ( 'NONE', *, *, #33386, .T. ) ;
#16289=CLOSED_SHELL ( 'NONE', ( #41860, #6726, #17416, #32462, #27067, #4351, #46629, #49747, #3928, #2692, #12943, #38317, #33208, #44374, #43689, #20363, #21584, #47421, #48196, #14705, #40003, #15502, #48388, #12089, #22410, #44056, #27471, #2287, #11175, #20483, #26212, #38110, #30945, #23651, #19328, #18730, #22113, #49015, #46681, #1376, #47790, #16478 ) ) ;
#16321=AXIS2_PLACEMENT_3D ( 'NONE', #4661, #19791, #20050 ) ;
#16325=VECTOR ( 'NONE', #15663, 1000.000000000000000 ) ;
#16352=AXIS2_PLACEMENT_3D ( 'NONE', #15038, #46041, #45793 ) ;
#16450=PRODUCT_CONTEXT ( 'NONE', #32208, 'mechanical' ) ;
#16478=ADVANCED_FACE ( 'NONE', ( #19195 ), #15111, .T. ) ;
#16491=DIRECTION ( 'NONE',  ( 0.000000000000000000, 0.000000000000000000, -1.000000000000000000 ) ) ;
#16596=ORIENTED_EDGE ( 'NONE', *, *, #13563, .F. ) ;
#16614=DIRECTION ( 'NONE',  ( -1.000000000000000000, 0.000000000000000000, 0.000000000000000000 ) ) ;
#16671=ORIENTED_EDGE ( 'NONE', *, *, #33326, .T. ) ;
#16690=CARTESIAN_POINT ( 'NONE',  ( -165.3973046169136012, 54.43801056904003133, -17.65743994998275213 ) ) ;
#16709=DIRECTION ( 'NONE',  ( 1.000000000000000000, -0.000000000000000000, -0.000000000000000000 ) ) ;
#16731=PLANE ( 'NONE',  #41345 ) ;
#16879=VECTOR ( 'NONE', #36327, 1000.000000000000000 ) ;
#16901=CARTESIAN_POINT ( 'NONE',  ( 154.1026953830863420, 103.9380105690400597, -17.65743994998277699 ) ) ;
#16928=ORIENTED_EDGE ( 'NONE', *, *, #10726, .F. ) ;
#16934=EDGE_CURVE ( 'NONE', #50336, #46082, #4518, .T. ) ;
#16935=DIRECTION ( 'NONE',  ( -0.8637789008984334549, 0.000000000000000000, 0.5038710255240862468 ) ) ;
#16951=VECTOR ( 'NONE', #48249, 1000.000000000000000 ) ;
#16952=VERTEX_POINT ( 'NONE', #15812 ) ;
#17061=DIRECTION ( 'NONE',  ( 0.000000000000000000, -1.000000000000000000, 0.000000000000000000 ) ) ;
#17117=VECTOR ( 'NONE', #40009, 1000.000000000000000 ) ;
#17149=DIRECTION ( 'NONE',  ( 0.000000000000000000, 1.000000000000000000, 0.000000000000000000 ) ) ;
#17181=CARTESIAN_POINT ( 'NONE',  ( -5.647304616913629616, 296.6525076104601339, 145.3277671506088780 ) ) ;
#17238=CARTESIAN_POINT ( 'NONE',  ( -5.647304616913629616, 2.688010569040066411, 741.9425600500172777 ) ) ;
#17276=VECTOR ( 'NONE', #46169, 1000.000000000000114 ) ;
#17300=DIRECTION ( 'NONE',  ( -0.000000000000000000, -0.000000000000000000, 1.000000000000000000 ) ) ;
#17318=ORIENTED_EDGE ( 'NONE', *, *, #23988, .T. ) ;
#17350=EDGE_CURVE ( 'NONE', #25227, #42832, #42179, .T. ) ;
#17386=CARTESIAN_POINT ( 'NONE',  ( 154.1026953830863420, 103.9380105690400597, -17.65743994998277699 ) ) ;
#17416=ADVANCED_FACE ( 'NONE', ( #46753 ), #46500, .F. ) ;
#17516=LINE ( 'NONE', #43690, #40890 ) ;
#17517=DIRECTION ( 'NONE',  ( 0.000000000000000000, -0.4027858274925602000, -0.9152942571496522906 ) ) ;
#17555=CARTESIAN_POINT ( 'NONE',  ( -310.0878471510133068, -227.3959007404658337, 296.3011729072028402 ) ) ;
#17600=VERTEX_POINT ( 'NONE', #36792 ) ;
#17636=CARTESIAN_POINT ( 'NONE',  ( 370.7621192902014968, -97.72914955339486198, -17.31629813440246579 ) ) ;
#17681=VECTOR ( 'NONE', #8166, 1000.000000000000000 ) ;
#17684=FACE_OUTER_BOUND ( 'NONE', #30910, .T. ) ;
#17729=LINE ( 'NONE', #10283, #44511 ) ;
#17763=DIRECTION ( 'NONE',  ( 0.000000000000000000, 0.3790464617558786942, -0.9253776417389547593 ) ) ;
#17770=DIRECTION ( 'NONE',  ( 0.000000000000000000, 0.000000000000000000, -1.000000000000000000 ) ) ;
#17774=PLANE ( 'NONE',  #19285 ) ;
#17784=ORIENTED_EDGE ( 'NONE', *, *, #29412, .T. ) ;
#17795=DIRECTION ( 'NONE',  ( -0.9928768384869219865, 0.000000000000000000, -0.1191452206184307888 ) ) ;
#17817=CARTESIAN_POINT ( 'NONE',  ( -165.3973046169136012, -98.56198943095992604, -17.65743994998275213 ) ) ;
#17822=CARTESIAN_POINT ( 'NONE',  ( -165.3973046169136012, 103.9380105690400597, 22.84256005001721945 ) ) ;
#17825=EDGE_CURVE ( 'NONE', #38528, #32226, #43139, .T. ) ;
#17858=EDGE_CURVE ( 'NONE', #20963, #12440, #32102, .T. ) ;
#17866=EDGE_LOOP ( 'NONE', ( #11328, #24462, #21106, #9643 ) ) ;
#17925=EDGE_LOOP ( 'NONE', ( #49517, #279, #22847, #12680, #6972, #47225 ) ) ;
#17941=VECTOR ( 'NONE', #32167, 999.9999999999998863 ) ;
#17952=VECTOR ( 'NONE', #34975, 1000.000000000000000 ) ;
#17973=EDGE_LOOP ( 'NONE', ( #15807, #20718, #48169, #15998, #38955 ) ) ;
#18106=CARTESIAN_POINT ( 'NONE',  ( -164.4973046169135955, -61.66198943095990614, -17.65743994998277699 ) ) ;
#18121=ORIENTED_EDGE ( 'NONE', *, *, #18380, .T. ) ;
#18162=VECTOR ( 'NONE', #19850, 1000.000000000000000 ) ;
#18195=VECTOR ( 'NONE', #41146, 1000.000000000000227 ) ;
#18220=CARTESIAN_POINT ( 'NONE',  ( -164.4973046169135955, -98.56198943095992604, -17.65743994998277699 ) ) ;
#18255=FACE_OUTER_BOUND ( 'NONE', #22595, .T. ) ;
#18327=CARTESIAN_POINT ( 'NONE',  ( 195.9526953830863079, -154.8119894309599260, 472.5992458228020610 ) ) ;
#18380=EDGE_CURVE ( 'NONE', #30787, #40281, #18830, .T. ) ;
#18575=VERTEX_POINT ( 'NONE', #5973 ) ;
#18588=ORIENTED_EDGE ( 'NONE', *, *, #33547, .T. ) ;
#18625=ORIENTED_EDGE ( 'NONE', *, *, #46179, .T. ) ;
#18677=EDGE_LOOP ( 'NONE', ( #38077, #22774, #31187, #33069, #50211 ) ) ;
#18728=DIRECTION ( 'NONE',  ( 0.000000000000000000, 1.000000000000000000, 0.000000000000000000 ) ) ;
#18730=ADVANCED_FACE ( 'NONE', ( #15195 ), #2377, .F. ) ;
#18738=PLANE ( 'NONE',  #14455 ) ;
#18759=VECTOR ( 'NONE', #332, 1000.000000000000000 ) ;
#18773=LINE ( 'NONE', #38315, #48238 ) ;
#18830=LINE ( 'NONE', #49338, #23312 ) ;
#18936=DIRECTION ( 'NONE',  ( -1.000000000000000000, -0.000000000000000000, -0.000000000000000000 ) ) ;
#18949=DIRECTION ( 'NONE',  ( -0.000000000000000000, 0.000000000000000000, 1.000000000000000000 ) ) ;
#18989=LINE ( 'NONE', #17555, #18195 ) ;
#19001=LINE ( 'NONE', #11320, #17276 ) ;
#19060=EDGE_LOOP ( 'NONE', ( #28434, #29559, #39359, #11246, #13205, #8217, #16236, #2909, #35908, #4434 ) ) ;
#19073=ORIENTED_EDGE ( 'NONE', *, *, #27060, .F. ) ;
#19167=DIRECTION ( 'NONE',  ( 0.000000000000000000, -0.000000000000000000, 1.000000000000000000 ) ) ;
#19195=FACE_OUTER_BOUND ( 'NONE', #3023, .T. ) ;
#19234=AXIS2_PLACEMENT_3D ( 'NONE', #10078, #2862, #50029 ) ;
#19235=ORIENTED_EDGE ( 'NONE', *, *, #10019, .T. ) ;
#19272=AXIS2_PLACEMENT_3D ( 'NONE', #38892, #19369, #35052 ) ;
#19279=VECTOR ( 'NONE', #25161, 1000.000000000000114 ) ;
#19285=AXIS2_PLACEMENT_3D ( 'NONE', #10334, #33934, #13406 ) ;
#19328=ADVANCED_FACE ( 'NONE', ( #5588 ), #13538, .T. ) ;
#19335=EDGE_CURVE ( 'NONE', #38770, #22476, #44823, .T. ) ;
#19348=ORIENTED_EDGE ( 'NONE', *, *, #20076, .F. ) ;
#19352=EDGE_CURVE ( 'NONE', #29505, #20059, #44078, .T. ) ;
#19369=DIRECTION ( 'NONE',  ( 0.000000000000000000, -1.000000000000000000, 0.000000000000000000 ) ) ;
#19376=ORIENTED_EDGE ( 'NONE', *, *, #4571, .T. ) ;
#19441=CARTESIAN_POINT ( 'NONE',  ( -5.647304616913629616, 295.8217383796908848, 144.9816133044550668 ) ) ;
#19633=VERTEX_POINT ( 'NONE', #48339 ) ;
#19685=VECTOR ( 'NONE', #32091, 1000.000000000000000 ) ;
#19693=LINE ( 'NONE', #23801, #36963 ) ;
#19694=EDGE_CURVE ( 'NONE', #44652, #48624, #4773, .T. ) ;
#19736=DIRECTION ( 'NONE',  ( 0.000000000000000000, 1.000000000000000000, 0.000000000000000000 ) ) ;
#19791=DIRECTION ( 'NONE',  ( -1.000000000000000000, 0.000000000000000000, 0.000000000000000000 ) ) ;
#19803=CARTESIAN_POINT ( 'NONE',  ( -50.64730461691362962, 47.68801056904006685, 742.8425600500171413 ) ) ;
#19813=EDGE_CURVE ( 'NONE', #357, #22708, #39474, .T. ) ;
#19850=DIRECTION ( 'NONE',  ( 0.000000000000000000, -0.000000000000000000, 1.000000000000000000 ) ) ;
#19915=AXIS2_PLACEMENT_3D ( 'NONE', #16091, #11733, #27899 ) ;
#19916=DIRECTION ( 'NONE',  ( 0.000000000000000000, 1.000000000000000000, 0.000000000000000000 ) ) ;
#19923=EDGE_CURVE ( 'NONE', #38528, #14628, #25828, .T. ) ;
#19977=DIRECTION ( 'NONE',  ( -0.000000000000000000, -0.000000000000000000, 1.000000000000000000 ) ) ;
#19989=DIRECTION ( 'NONE',  ( -0.5038710255240859137, 0.000000000000000000, 0.8637789008984335659 ) ) ;
#19991=VECTOR ( 'NONE', #12557, 1000.000000000000000 ) ;
#20001=ORIENTED_EDGE ( 'NONE', *, *, #45223, .T. ) ;
#20050=DIRECTION ( 'NONE',  ( 0.000000000000000000, 0.000000000000000000, 1.000000000000000000 ) ) ;
#20059=VERTEX_POINT ( 'NONE', #24768 ) ;
#20076=EDGE_CURVE ( 'NONE', #12440, #20059, #27609, .T. ) ;
#20088=VERTEX_POINT ( 'NONE', #43988 ) ;
#20104=VECTOR ( 'NONE', #28875, 1000.000000000000114 ) ;
#20157=ORIENTED_EDGE ( 'NONE', *, *, #30569, .T. ) ;
#20174=LINE ( 'NONE', #28391, #3208 ) ;
#20179=DIRECTION ( 'NONE',  ( 0.000000000000000000, -0.3790464617558786942, 0.9253776417389547593 ) ) ;
#20349=ORIENTED_EDGE ( 'NONE', *, *, #30936, .F. ) ;
#20363=ADVANCED_FACE ( 'NONE', ( #49810 ), #7797, .T. ) ;
#20433=VECTOR ( 'NONE', #28839, 1000.000000000000000 ) ;
#20466=CARTESIAN_POINT ( 'NONE',  ( -5.647304616913629616, -154.8119894309598408, 472.8425600500173118 ) ) ;
#20471=LINE ( 'NONE', #7677, #12017 ) ;
#20483=ADVANCED_FACE ( 'NONE', ( #28294 ), #12632, .F. ) ;
#20484=VECTOR ( 'NONE', #45762, 1000.000000000000000 ) ;
#20528=VECTOR ( 'NONE', #44237, 1000.000000000000000 ) ;
#20550=LINE ( 'NONE', #29762, #33050 ) ;
#20577=ORIENTED_EDGE ( 'NONE', *, *, #17350, .F. ) ;
#20628=AXIS2_PLACEMENT_3D ( 'NONE', #28040, #28547, #43672 ) ;
#20659=VERTEX_POINT ( 'NONE', #22609 ) ;
#20718=ORIENTED_EDGE ( 'NONE', *, *, #19923, .F. ) ;
#20777=ORIENTED_EDGE ( 'NONE', *, *, #34938, .T. ) ;
#20809=LINE ( 'NONE', #33146, #23787 ) ;
#20955=DIRECTION ( 'NONE',  ( 0.000000000000000000, -1.000000000000000000, 1.822804496942679766E-16 ) ) ;
#20963=VERTEX_POINT ( 'NONE', #2481 ) ;
#20975=CARTESIAN_POINT ( 'NONE',  ( -50.13037131770489907, 47.08801056904012228, 741.9425600500172777 ) ) ;
#21106=ORIENTED_EDGE ( 'NONE', *, *, #33550, .F. ) ;
#21263=ORIENTED_EDGE ( 'NONE', *, *, #29896, .F. ) ;
#21295=DIRECTION ( 'NONE',  ( 0.000000000000000000, 1.000000000000000000, 0.000000000000000000 ) ) ;
#21328=FACE_OUTER_BOUND ( 'NONE', #4617, .T. ) ;
#21351=CARTESIAN_POINT ( 'NONE',  ( 370.7621192902014968, -98.56198943095992604, -17.65743994998275213 ) ) ;
#21420=VECTOR ( 'NONE', #22414, 999.9999999999998863 ) ;
#21437=PLANE ( 'NONE',  #39369 ) ;
#21517=CARTESIAN_POINT ( 'NONE',  ( -352.5903097982607051, 2.688010569040066411, 225.2259797391364771 ) ) ;
#21584=ADVANCED_FACE ( 'NONE', ( #40852 ), #5701, .T. ) ;
#21642=VERTEX_POINT ( 'NONE', #26729 ) ;
#21672=CARTESIAN_POINT ( 'NONE',  ( 154.1026953830863420, -98.56198943095992604, 22.84256005001721945 ) ) ;
#21849=CARTESIAN_POINT ( 'NONE',  ( -543.5890838333644979, 53.53801056904005407, -176.2581102438216192 ) ) ;
#22020=EDGE_CURVE ( 'NONE', #9657, #13193, #27427, .T. ) ;
#22038=EDGE_CURVE ( 'NONE', #3725, #18575, #20471, .T. ) ;
#22110=EDGE_CURVE ( 'NONE', #29505, #11397, #25593, .T. ) ;
#22113=ADVANCED_FACE ( 'NONE', ( #37418 ), #9686, .F. ) ;
#22178=ORIENTED_EDGE ( 'NONE', *, *, #48045, .F. ) ;
#22207=VECTOR ( 'NONE', #17795, 1000.000000000000227 ) ;
#22213=VECTOR ( 'NONE', #45765, 1000.000000000000114 ) ;
#22272=ORIENTED_EDGE ( 'NONE', *, *, #48045, .T. ) ;
#22326=EDGE_LOOP ( 'NONE', ( #35611, #49086, #8168, #47366 ) ) ;
#22342=CARTESIAN_POINT ( 'NONE',  ( 196.8526953830863135, 160.1880105690400171, 472.8425600500171981 ) ) ;
#22389=EDGE_CURVE ( 'NONE', #27616, #27480, #31928, .T. ) ;
#22410=ADVANCED_FACE ( 'NONE', ( #18255 ), #17774, .T. ) ;
#22414=DIRECTION ( 'NONE',  ( 0.000000000000000000, -0.3846153846153845812, -0.9230769230769231282 ) ) ;
#22476=VERTEX_POINT ( 'NONE', #48778 ) ;
#22574=MANIFOLD_SOLID_BREP ( 'Scale1', #16289 ) ;
#22590=EDGE_LOOP ( 'NONE', ( #31820, #19235, #36180, #43674 ) ) ;
#22595=EDGE_LOOP ( 'NONE', ( #30542, #8605, #24066, #47911, #9532, #25366 ) ) ;
#22609=CARTESIAN_POINT ( 'NONE',  ( -208.1473046169136296, 160.1880105690400171, 472.8425600500171981 ) ) ;
#22621=VERTEX_POINT ( 'NONE', #16690 ) ;
#22695=DIRECTION ( 'NONE',  ( 0.000000000000000000, -0.9230769230769231282, 0.3846153846153845812 ) ) ;
#22697=DIRECTION ( 'NONE',  ( 0.4740998230350172427, -0.3386427307392981256, -0.8127425537743157014 ) ) ;
#22698=EDGE_CURVE ( 'NONE', #20659, #34186, #43036, .T. ) ;
#22708=VERTEX_POINT ( 'NONE', #15602 ) ;
#22774=ORIENTED_EDGE ( 'NONE', *, *, #30936, .T. ) ;
#22795=CARTESIAN_POINT ( 'NONE',  ( 195.9157620838774676, 159.2880105690400399, 472.6625600500173050 ) ) ;
#22847=ORIENTED_EDGE ( 'NONE', *, *, #28503, .T. ) ;
#22848=DIRECTION ( 'NONE',  ( -0.000000000000000000, -0.000000000000000000, -1.000000000000000000 ) ) ;
#22852=FACE_OUTER_BOUND ( 'NONE', #27015, .T. ) ;
#22856=CARTESIAN_POINT ( 'NONE',  ( -543.3973046169135159, 54.43801056904003133, -177.1374399499827916 ) ) ;
#22910=ORIENTED_EDGE ( 'NONE', *, *, #28399, .T. ) ;
#23001=VERTEX_POINT ( 'NONE', #38707 ) ;
#23017=EDGE_CURVE ( 'NONE', #28855, #19633, #35633, .T. ) ;
#23100=LINE ( 'NONE', #26953, #15758 ) ;
#23127=( LENGTH_UNIT ( ) NAMED_UNIT ( * ) SI_UNIT ( .MILLI., .METRE. ) );
#23209=PLANE ( 'NONE',  #19272 ) ;
#23248=VECTOR ( 'NONE', #13030, 1000.000000000000000 ) ;
#23312=VECTOR ( 'NONE', #14745, 1000.000000000000000 ) ;
#23382=ORIENTED_EDGE ( 'NONE', *, *, #43549, .F. ) ;
#23433=CARTESIAN_POINT ( 'NONE',  ( 154.1026953830863420, -97.66198943095992036, -17.48025818148969890 ) ) ;
#23458=DIRECTION ( 'NONE',  ( 0.4740998230350172427, 0.3386427307392981256, -0.8127425537743157014 ) ) ;
#23565=ORIENTED_EDGE ( 'NONE', *, *, #17858, .F. ) ;
#23577=DIRECTION ( 'NONE',  ( 0.000000000000000000, -0.000000000000000000, 1.000000000000000000 ) ) ;
#23635=ORIENTED_EDGE ( 'NONE', *, *, #27935, .T. ) ;
#23651=ADVANCED_FACE ( 'NONE', ( #22852 ), #18738, .T. ) ;
#23771=CARTESIAN_POINT ( 'NONE',  ( 153.2026953830863647, -97.66198943095992036, 23.74256005001722158 ) ) ;
#23787=VECTOR ( 'NONE', #16709, 1000.000000000000000 ) ;
#23793=VECTOR ( 'NONE', #30964, 1000.000000000000000 ) ;
#23801=CARTESIAN_POINT ( 'NONE',  ( 298.7932379171858770, -227.3959007404659474, 296.3011729072026696 ) ) ;
#23837=LINE ( 'NONE', #43064, #1073 ) ;
#23921=CARTESIAN_POINT ( 'NONE',  ( -5.647304616913629616, 2.688010569040066411, 23.74256005001722158 ) ) ;
#23927=ORIENTED_EDGE ( 'NONE', *, *, #44105, .T. ) ;
#23988=EDGE_CURVE ( 'NONE', #25227, #7200, #30500, .T. ) ;
#24053=FACE_OUTER_BOUND ( 'NONE', #18677, .T. ) ;
#24066=ORIENTED_EDGE ( 'NONE', *, *, #38775, .T. ) ;
#24071=CARTESIAN_POINT ( 'NONE',  ( -164.4973046169135955, -98.56198943095992604, -18.45589678844777382 ) ) ;
#24087=VECTOR ( 'NONE', #19977, 1000.000000000000000 ) ;
#24139=ORIENTED_EDGE ( 'NONE', *, *, #24660, .T. ) ;
#24202=CARTESIAN_POINT ( 'NONE',  ( -351.8129087874521588, 2.688010569040066411, 224.7724958161647635 ) ) ;
#24219=DIRECTION ( 'NONE',  ( -0.9928768384869219865, 0.000000000000000000, -0.1191452206184307749 ) ) ;
#24240=ORIENTED_EDGE ( 'NONE', *, *, #37620, .F. ) ;
#24462=ORIENTED_EDGE ( 'NONE', *, *, #44466, .T. ) ;
#24472=CARTESIAN_POINT ( 'NONE',  ( 154.1026953830863420, 103.0380105690400683, -17.65743994998277699 ) ) ;
#24539=DIRECTION ( 'NONE',  ( 0.000000000000000000, 1.000000000000000000, 0.000000000000000000 ) ) ;
#24599=CARTESIAN_POINT ( 'NONE',  ( -543.5050241616419271, 53.53801056904005407, -176.2397770772458898 ) ) ;
#24602=CARTESIAN_POINT ( 'NONE',  ( -310.0878471510133068, 232.7719218785459816, 296.3011729072028402 ) ) ;
#24626=LINE ( 'NONE', #12305, #4135 ) ;
#24658=SHAPE_DEFINITION_REPRESENTATION ( #10572, #31369 ) ;
#24660=EDGE_CURVE ( 'NONE', #30282, #26345, #40677, .T. ) ;
#24686=ORIENTED_EDGE ( 'NONE', *, *, #17858, .T. ) ;
#24768=CARTESIAN_POINT ( 'NONE',  ( -207.2103713177049258, 159.2880105690400399, 472.6625600500171345 ) ) ;
#24809=LINE ( 'NONE', #2213, #39029 ) ;
#24812=ORIENTED_EDGE ( 'NONE', *, *, #23017, .F. ) ;
#24848=FACE_BOUND ( 'NONE', #49054, .T. ) ;
#24962=ORIENTED_EDGE ( 'NONE', *, *, #42525, .T. ) ;
#24976=CARTESIAN_POINT ( 'NONE',  ( -164.4973046169135102, 103.1142457376053727, -17.29493270523947501 ) ) ;
#24993=CARTESIAN_POINT ( 'NONE',  ( -556.7900739183570522, -61.66198943095990614, -65.53102910462104091 ) ) ;
#25046=VECTOR ( 'NONE', #30674, 1000.000000000000227 ) ;
#25055=CARTESIAN_POINT ( 'NONE',  ( -165.3973046169136012, 54.43801056904003133, -17.65743994998275213 ) ) ;
#25134=DIRECTION ( 'NONE',  ( 0.5038710255240862468, 0.000000000000000000, 0.8637789008984334549 ) ) ;
#25151=LINE ( 'NONE', #37473, #9190 ) ;
#25160=DIRECTION ( 'NONE',  ( 0.9928768384869219865, 0.000000000000000000, 0.1191452206184307749 ) ) ;
#25161=DIRECTION ( 'NONE',  ( 0.4740998230350171871, 0.3386427307392981256, -0.8127425537743158124 ) ) ;
#25199=CARTESIAN_POINT ( 'NONE',  ( -165.3973046169136012, -98.56198943095992604, 22.84256005001721945 ) ) ;
#25216=CARTESIAN_POINT ( 'NONE',  ( -207.2473046169136808, -154.8119894309599260, 470.5025600500171095 ) ) ;
#25217=CARTESIAN_POINT ( 'NONE',  ( -207.2473046169136808, -154.8119894309599260, 472.8425600500171981 ) ) ;
#25226=DIRECTION ( 'NONE',  ( -0.9928768384869219865, 0.000000000000000000, -0.1191452206184307888 ) ) ;
#25227=VERTEX_POINT ( 'NONE', #3817 ) ;
#25240=LINE ( 'NONE', #5732, #20433 ) ;
#25317=CARTESIAN_POINT ( 'NONE',  ( -207.2473046169136808, 159.2880105690400399, 472.8425600500171981 ) ) ;
#25346=CARTESIAN_POINT ( 'NONE',  ( -5.647304616913629616, 2.688010569040066411, 22.84256005001721945 ) ) ;
#25366=ORIENTED_EDGE ( 'NONE', *, *, #19923, .T. ) ;
#25376=LINE ( 'NONE', #29475, #28703 ) ;
#25392=VERTEX_POINT ( 'NONE', #40989 ) ;
#25574=VERTEX_POINT ( 'NONE', #7878 ) ;
#25593=LINE ( 'NONE', #13270, #39868 ) ;
#25611=CARTESIAN_POINT ( 'NONE',  ( 154.1026953830863420, 103.0380105690400683, -17.46817021067766973 ) ) ;
#25688=LINE ( 'NONE', #37509, #33281 ) ;
#25689=VECTOR ( 'NONE', #30786, 1000.000000000000000 ) ;
#25767=VERTEX_POINT ( 'NONE', #48833 ) ;
#25828=LINE ( 'NONE', #25317, #7879 ) ;
#25859=VECTOR ( 'NONE', #46321, 1000.000000000000000 ) ;
#26023=ORIENTED_EDGE ( 'NONE', *, *, #4639, .T. ) ;
#26038=CARTESIAN_POINT ( 'NONE',  ( -208.1473046169136580, -154.8119894309599260, 22.84256005001721945 ) ) ;
#26188=DIRECTION ( 'NONE',  ( -0.000000000000000000, 0.000000000000000000, 1.000000000000000000 ) ) ;
#26212=ADVANCED_FACE ( 'NONE', ( #45440 ), #45187, .F. ) ;
#26215=DIRECTION ( 'NONE',  ( 0.000000000000000000, 0.000000000000000000, -1.000000000000000000 ) ) ;
#26246=VECTOR ( 'NONE', #27629, 999.9999999999998863 ) ;
#26270=CARTESIAN_POINT ( 'NONE',  ( 154.1026953830863420, -98.56198943095992604, -17.65743994998275213 ) ) ;
#26345=VERTEX_POINT ( 'NONE', #7497 ) ;
#26471=( NAMED_UNIT ( * ) SI_UNIT ( $, .STERADIAN. ) SOLID_ANGLE_UNIT ( ) );
#26493=ORIENTED_EDGE ( 'NONE', *, *, #9799, .T. ) ;
#26547=PRODUCT_DEFINITION ( 'UNKNOWN', '', #49539, #31917 ) ;
#26563=CARTESIAN_POINT ( 'NONE',  ( -50.64730461691362962, 47.68801056904006685, 742.8425600500171413 ) ) ;
#26672=CARTESIAN_POINT ( 'NONE',  ( -164.4973046169135955, -97.66198943095992036, -17.65743994998277699 ) ) ;
#26729=CARTESIAN_POINT ( 'NONE',  ( -165.3973046169136012, 70.03596893647589638, -94.69675437945477370 ) ) ;
#26748=CARTESIAN_POINT ( 'NONE',  ( -543.3973046169135159, -62.56198943095993315, -177.1374399499827916 ) ) ;
#26754=LINE ( 'NONE', #50557, #18759 ) ;
#26783=CARTESIAN_POINT ( 'NONE',  ( 195.9526953830863079, -290.4457172416107937, 144.9816133044550668 ) ) ;
#26887=DIRECTION ( 'NONE',  ( 0.000000000000000000, -0.3846153846153844702, 0.9230769230769231282 ) ) ;
#26897=ORIENTED_EDGE ( 'NONE', *, *, #5165, .F. ) ;
#26903=CARTESIAN_POINT ( 'NONE',  ( -5.647304616913629616, 47.08801056904012228, 741.9425600500172777 ) ) ;
#26940=ORIENTED_EDGE ( 'NONE', *, *, #22110, .F. ) ;
#26953=CARTESIAN_POINT ( 'NONE',  ( -165.3973046169136012, 103.9380105690400597, -17.65743994998277699 ) ) ;
#27015=EDGE_LOOP ( 'NONE', ( #4427, #6768, #48270, #24240, #34043, #24962 ) ) ;
#27025=DIRECTION ( 'NONE',  ( 0.000000000000000000, 0.9152942571496521795, -0.4027858274925601445 ) ) ;
#27060=EDGE_CURVE ( 'NONE', #7200, #20659, #46272, .T. ) ;
#27067=ADVANCED_FACE ( 'NONE', ( #7575 ), #23209, .F. ) ;
#27104=UNCERTAINTY_MEASURE_WITH_UNIT (LENGTH_MEASURE( 1.000000000000000082E-05 ), #23127, 'distance_accuracy_value', 'NONE');
#27207=CARTESIAN_POINT ( 'NONE',  ( -164.4973046169135955, 103.0380105690400683, 23.74256005001722158 ) ) ;
#27228=AXIS2_PLACEMENT_3D ( 'NONE', #27254, #7761, #15696 ) ;
#27254=CARTESIAN_POINT ( 'NONE',  ( -5.647304616913629616, -291.2764864723799860, 145.3277671506088780 ) ) ;
#27261=VECTOR ( 'NONE', #615, 1000.000000000000000 ) ;
#27276=ORIENTED_EDGE ( 'NONE', *, *, #36565, .T. ) ;
#27392=ORIENTED_EDGE ( 'NONE', *, *, #23988, .F. ) ;
#27427=LINE ( 'NONE', #39999, #7067 ) ;
#27471=ADVANCED_FACE ( 'NONE', ( #31386, #28025 ), #42901, .F. ) ;
#27480=VERTEX_POINT ( 'NONE', #3911 ) ;
#27514=VECTOR ( 'NONE', #18936, 1000.000000000000000 ) ;
#27524=EDGE_CURVE ( 'NONE', #13193, #27616, #29035, .T. ) ;
#27564=CARTESIAN_POINT ( 'NONE',  ( -165.3973046169136012, -67.00570555996102939, -94.69675437945474528 ) ) ;
#27609=LINE ( 'NONE', #32216, #16879 ) ;
#27616=VERTEX_POINT ( 'NONE', #48231 ) ;
#27621=ORIENTED_EDGE ( 'NONE', *, *, #14417, .T. ) ;
#27629=DIRECTION ( 'NONE',  ( 0.1191452206184307611, 0.000000000000000000, -0.9928768384869220975 ) ) ;
#27787=AXIS2_PLACEMENT_3D ( 'NONE', #12845, #47953, #25160 ) ;
#27899=DIRECTION ( 'NONE',  ( 0.000000000000000000, -0.000000000000000000, 1.000000000000000000 ) ) ;
#27935=EDGE_CURVE ( 'NONE', #33351, #17600, #29229, .T. ) ;
#28025=FACE_OUTER_BOUND ( 'NONE', #30301, .T. ) ;
#28040=CARTESIAN_POINT ( 'NONE',  ( 154.1026953830863420, -98.56198943095992604, -17.65743994998277699 ) ) ;
#28042=ORIENTED_EDGE ( 'NONE', *, *, #9209, .T. ) ;
#28060=DIRECTION ( 'NONE',  ( 1.000000000000000000, 0.000000000000000000, 0.000000000000000000 ) ) ;
#28081=EDGE_CURVE ( 'NONE', #17600, #15132, #11681, .T. ) ;
#28091=DIRECTION ( 'NONE',  ( 1.000000000000000000, 0.000000000000000000, 0.000000000000000000 ) ) ;
#28221=EDGE_LOOP ( 'NONE', ( #36827, #44500, #26897, #28911 ) ) ;
#28294=FACE_OUTER_BOUND ( 'NONE', #50219, .T. ) ;
#28391=CARTESIAN_POINT ( 'NONE',  ( 196.8526953830863135, -154.8119894309599260, 22.84256005001721945 ) ) ;
#28399=EDGE_CURVE ( 'NONE', #36023, #25392, #37081, .T. ) ;
#28434=ORIENTED_EDGE ( 'NONE', *, *, #28081, .F. ) ;
#28444=DIRECTION ( 'NONE',  ( 0.000000000000000000, -1.000000000000000000, 0.000000000000000000 ) ) ;
#28480=VERTEX_POINT ( 'NONE', #7016 ) ;
#28503=EDGE_CURVE ( 'NONE', #23001, #14108, #38336, .T. ) ;
#28547=DIRECTION ( 'NONE',  ( 0.000000000000000000, 1.000000000000000000, 0.000000000000000000 ) ) ;
#28592=ORIENTED_EDGE ( 'NONE', *, *, #50581, .T. ) ;
#28703=VECTOR ( 'NONE', #45094, 1000.000000000000114 ) ;
#28740=DIRECTION ( 'NONE',  ( 0.000000000000000000, 0.000000000000000000, 1.000000000000000000 ) ) ;
#28754=ORIENTED_EDGE ( 'NONE', *, *, #28081, .T. ) ;
#28773=VECTOR ( 'NONE', #30406, 1000.000000000000000 ) ;
#28777=CARTESIAN_POINT ( 'NONE',  ( -164.4973046169135955, 53.53801056904001854, -17.65743994998277699 ) ) ;
#28799=EDGE_CURVE ( 'NONE', #42832, #29402, #30561, .T. ) ;
#28817=LINE ( 'NONE', #24976, #46523 ) ;
#28839=DIRECTION ( 'NONE',  ( -1.000000000000000000, 0.000000000000000000, 0.000000000000000000 ) ) ;
#28855=VERTEX_POINT ( 'NONE', #2583 ) ;
#28875=DIRECTION ( 'NONE',  ( -0.9928768384869219865, 0.000000000000000000, -0.1191452206184307749 ) ) ;
#28904=LINE ( 'NONE', #44523, #10343 ) ;
#28911=ORIENTED_EDGE ( 'NONE', *, *, #34999, .F. ) ;
#29018=CARTESIAN_POINT ( 'NONE',  ( -207.2473046169136808, 159.2880105690400399, 472.5992458228020610 ) ) ;
#29035=LINE ( 'NONE', #21849, #14371 ) ;
#29125=VECTOR ( 'NONE', #36673, 999.9999999999998863 ) ;
#29185=AXIS2_PLACEMENT_3D ( 'NONE', #24202, #39863, #8048 ) ;
#29229=LINE ( 'NONE', #10663, #1314 ) ;
#29251=CARTESIAN_POINT ( 'NONE',  ( 195.9526953830863079, 2.688010569040066411, 23.74256005001722158 ) ) ;
#29263=DIRECTION ( 'NONE',  ( 0.000000000000000000, 1.000000000000000000, -1.822804496942680012E-16 ) ) ;
#29304=ORIENTED_EDGE ( 'NONE', *, *, #9516, .F. ) ;
#29391=CARTESIAN_POINT ( 'NONE',  ( -543.3973046169135159, 54.43801056904003133, -177.1374399499827916 ) ) ;
#29402=VERTEX_POINT ( 'NONE', #29421 ) ;
#29408=LINE ( 'NONE', #18106, #33605 ) ;
#29409=DIRECTION ( 'NONE',  ( 0.000000000000000000, -1.822804496942679766E-16, -1.000000000000000000 ) ) ;
#29412=EDGE_CURVE ( 'NONE', #33082, #21642, #37150, .T. ) ;
#29421=CARTESIAN_POINT ( 'NONE',  ( 196.8526953830863135, 160.1880105690400171, 22.84256005001721945 ) ) ;
#29459=DIRECTION ( 'NONE',  ( 0.000000000000000000, 0.000000000000000000, 1.000000000000000000 ) ) ;
#29475=CARTESIAN_POINT ( 'NONE',  ( -543.5890838333644979, -61.66198943095990614, -176.2581102438216192 ) ) ;
#29494=VECTOR ( 'NONE', #30731, 1000.000000000000000 ) ;
#29504=LINE ( 'NONE', #29251, #14981 ) ;
#29505=VERTEX_POINT ( 'NONE', #20975 ) ;
#29559=ORIENTED_EDGE ( 'NONE', *, *, #8894, .T. ) ;
#29563=SHAPE_REPRESENTATION_RELATIONSHIP ( 'NONE' , 'NONE' ,  #31369, #36305 ) ;
#29625=LINE ( 'NONE', #26038, #39789 ) ;
#29635=EDGE_CURVE ( 'NONE', #1211, #16952, #12885, .T. ) ;
#29639=LINE ( 'NONE', #18327, #17952 ) ;
#29708=LINE ( 'NONE', #25611, #10079 ) ;
#29762=CARTESIAN_POINT ( 'NONE',  ( 153.2026953830863647, 103.0380105690400683, -17.65743994998277699 ) ) ;
#29768=LINE ( 'NONE', #36999, #15507 ) ;
#29828=CARTESIAN_POINT ( 'NONE',  ( 340.5182995536247859, 2.688010569040066411, 224.7724958161645077 ) ) ;
#29853=ORIENTED_EDGE ( 'NONE', *, *, #43053, .F. ) ;
#29869=EDGE_LOOP ( 'NONE', ( #46781, #2751, #3758, #34579, #2832, #29997 ) ) ;
#29896=EDGE_CURVE ( 'NONE', #11397, #31874, #35681, .T. ) ;
#29957=STYLED_ITEM('',(#50782),#22574);
#29997=ORIENTED_EDGE ( 'NONE', *, *, #29412, .F. ) ;
#30098=DIRECTION ( 'NONE',  ( 0.000000000000000000, 0.000000000000000000, -1.000000000000000000 ) ) ;
#30282=VERTEX_POINT ( 'NONE', #44062 ) ;
#30301=EDGE_LOOP ( 'NONE', ( #20001, #5368, #702, #11836 ) ) ;
#30345=CARTESIAN_POINT ( 'NONE',  ( -165.3973046169136012, 103.9380105690400597, -17.65743994998277699 ) ) ;
#30357=VERTEX_POINT ( 'NONE', #10687 ) ;
#30377=CARTESIAN_POINT ( 'NONE',  ( 370.7621192902014968, 103.9380105690400597, -17.65743994998277699 ) ) ;
#30379=LINE ( 'NONE', #26783, #21420 ) ;
#30406=DIRECTION ( 'NONE',  ( 0.000000000000000000, -1.000000000000000000, 0.000000000000000000 ) ) ;
#30417=AXIS2_PLACEMENT_3D ( 'NONE', #17238, #13630, #36762 ) ;
#30436=PLANE ( 'NONE',  #16352 ) ;
#30478=LINE ( 'NONE', #49677, #15612 ) ;
#30490=DIRECTION ( 'NONE',  ( -0.000000000000000000, -0.000000000000000000, -1.000000000000000000 ) ) ;
#30497=VERTEX_POINT ( 'NONE', #23771 ) ;
#30500=LINE ( 'NONE', #6643, #27514 ) ;
#30514=VECTOR ( 'NONE', #19989, 1000.000000000000000 ) ;
#30542=ORIENTED_EDGE ( 'NONE', *, *, #46578, .F. ) ;
#30561=LINE ( 'NONE', #22342, #4605 ) ;
#30569=EDGE_CURVE ( 'NONE', #18575, #13303, #7103, .T. ) ;
#30674=DIRECTION ( 'NONE',  ( -0.4740998230350175202, 0.3386427307392980701, -0.8127425537743157014 ) ) ;
#30689=ORIENTED_EDGE ( 'NONE', *, *, #4264, .T. ) ;
#30731=DIRECTION ( 'NONE',  ( -1.000000000000000000, 0.000000000000000000, 0.000000000000000000 ) ) ;
#30750=FACE_OUTER_BOUND ( 'NONE', #2711, .T. ) ;
#30786=DIRECTION ( 'NONE',  ( 0.000000000000000000, 1.000000000000000000, -1.822804496942680012E-16 ) ) ;
#30787=VERTEX_POINT ( 'NONE', #21672 ) ;
#30823=VERTEX_POINT ( 'NONE', #17822 ) ;
#30910=EDGE_LOOP ( 'NONE', ( #14591, #26493, #19073, #27392 ) ) ;
#30922=LINE ( 'NONE', #38872, #18162 ) ;
#30936=EDGE_CURVE ( 'NONE', #28855, #9657, #35792, .T. ) ;
#30943=ORIENTED_EDGE ( 'NONE', *, *, #1719, .F. ) ;
#30945=ADVANCED_FACE ( 'NONE', ( #4211 ), #43201, .T. ) ;
#30964=DIRECTION ( 'NONE',  ( 1.000000000000000000, 0.000000000000000000, -0.000000000000000000 ) ) ;
#30967=ORIENTED_EDGE ( 'NONE', *, *, #4639, .F. ) ;
#31003=EDGE_CURVE ( 'NONE', #1016, #1211, #14153, .T. ) ;
#31004=FACE_OUTER_BOUND ( 'NONE', #42056, .T. ) ;
#31028=CARTESIAN_POINT ( 'NONE',  ( -5.647304616913629616, -61.66198943095990614, 22.84256005001721945 ) ) ;
#31034=EDGE_CURVE ( 'NONE', #12974, #42730, #28817, .T. ) ;
#31124=ORIENTED_EDGE ( 'NONE', *, *, #19694, .F. ) ;
#31187=ORIENTED_EDGE ( 'NONE', *, *, #22020, .T. ) ;
#31283=DIRECTION ( 'NONE',  ( 0.000000000000000000, 0.000000000000000000, 1.000000000000000000 ) ) ;
#31369=SHAPE_REPRESENTATION ( 'aluminum', ( #45486 ), #12706 ) ;
#31386=FACE_BOUND ( 'NONE', #22590, .T. ) ;
#31396=ORIENTED_EDGE ( 'NONE', *, *, #19813, .F. ) ;
#31435=CARTESIAN_POINT ( 'NONE',  ( -543.5050241616419271, 54.43801056904003133, -176.2397770772458898 ) ) ;
#31546=DIRECTION ( 'NONE',  ( 0.1191452206184307611, 0.000000000000000000, -0.9928768384869220975 ) ) ;
#31619=EDGE_LOOP ( 'NONE', ( #36755, #27621, #15697, #45457 ) ) ;
#31653=VECTOR ( 'NONE', #42219, 1000.000000000000000 ) ;
#31664=PLANE ( 'NONE',  #20628 ) ;
#31732=ORIENTED_EDGE ( 'NONE', *, *, #28399, .F. ) ;
#31752=ORIENTED_EDGE ( 'NONE', *, *, #6440, .F. ) ;
#31810=LINE ( 'NONE', #47388, #17117 ) ;
#31820=ORIENTED_EDGE ( 'NONE', *, *, #19694, .T. ) ;
#31856=VERTEX_POINT ( 'NONE', #49090 ) ;
#31874=VERTEX_POINT ( 'NONE', #7296 ) ;
#31917=PRODUCT_DEFINITION_CONTEXT ( 'detailed design', #37166, 'design' ) ;
#31920=ORIENTED_EDGE ( 'NONE', *, *, #24660, .F. ) ;
#31923=CARTESIAN_POINT ( 'NONE',  ( 0.000000000000000000, 0.000000000000000000, 0.000000000000000000 ) ) ;
#31928=LINE ( 'NONE', #12406, #41415 ) ;
#31953=CARTESIAN_POINT ( 'NONE',  ( 154.1026953830863420, 103.0380105690400683, 23.74256005001722158 ) ) ;
#31968=VECTOR ( 'NONE', #22697, 1000.000000000000000 ) ;
#32003=CARTESIAN_POINT ( 'NONE',  ( -207.2473046169136808, 159.2880105690400399, 23.74256005001722158 ) ) ;
#32064=DIRECTION ( 'NONE',  ( 1.000000000000000000, 0.000000000000000000, 0.000000000000000000 ) ) ;
#32086=FACE_OUTER_BOUND ( 'NONE', #36018, .T. ) ;
#32091=DIRECTION ( 'NONE',  ( 1.000000000000000000, 0.000000000000000000, 0.000000000000000000 ) ) ;
#32102=LINE ( 'NONE', #48456, #19279 ) ;
#32167=DIRECTION ( 'NONE',  ( 0.5038710255240862468, 0.000000000000000000, 0.8637789008984334549 ) ) ;
#32196=ORIENTED_EDGE ( 'NONE', *, *, #29635, .F. ) ;
#32208=APPLICATION_CONTEXT ( 'automotive_design' ) ;
#32216=CARTESIAN_POINT ( 'NONE',  ( -208.1473046169136580, 159.2880105690400399, 472.6625600500173050 ) ) ;
#32226=VERTEX_POINT ( 'NONE', #5715 ) ;
#32276=DIRECTION ( 'NONE',  ( -0.4740998230350175202, -0.3386427307392980701, -0.8127425537743157014 ) ) ;
#32284=EDGE_LOOP ( 'NONE', ( #50121, #2225, #2859, #4171, #14446, #29304 ) ) ;
#32320=CARTESIAN_POINT ( 'NONE',  ( -5.647304616913629616, -41.71198943095993172, 741.9425600500172777 ) ) ;
#32399=CARTESIAN_POINT ( 'NONE',  ( -5.647304616913629616, -154.8119894309599260, 23.74256005001722158 ) ) ;
#32462=ADVANCED_FACE ( 'NONE', ( #8516 ), #4152, .F. ) ;
#32477=CARTESIAN_POINT ( 'NONE',  ( -165.4943081650523027, 70.03596893647545585, -93.79675437945476801 ) ) ;
#32506=AXIS2_PLACEMENT_3D ( 'NONE', #17636, #5068, #33049 ) ;
#32509=EDGE_CURVE ( 'NONE', #14108, #33082, #29768, .T. ) ;
#32563=EDGE_CURVE ( 'NONE', #9657, #50336, #2068, .T. ) ;
#32613=CARTESIAN_POINT ( 'NONE',  ( -543.5050241616419271, -61.66198943095990614, -176.2397770772458898 ) ) ;
#32622=ORIENTED_EDGE ( 'NONE', *, *, #22389, .F. ) ;
#32729=VECTOR ( 'NONE', #49028, 1000.000000000000000 ) ;
#32748=EDGE_CURVE ( 'NONE', #30357, #30497, #31810, .T. ) ;
#32763=VECTOR ( 'NONE', #385, 1000.000000000000000 ) ;
#32827=EDGE_CURVE ( 'NONE', #40281, #30823, #6996, .T. ) ;
#32885=ORIENTED_EDGE ( 'NONE', *, *, #15510, .F. ) ;
#32937=CARTESIAN_POINT ( 'NONE',  ( -351.8129087874521588, 159.2880105690400399, 224.7724958161647635 ) ) ;
#32993=CARTESIAN_POINT ( 'NONE',  ( -165.2900739183569954, -61.66198943095990614, -18.55102910462098365 ) ) ;
#33049=DIRECTION ( 'NONE',  ( 0.000000000000000000, 0.3790464617558786942, -0.9253776417389547593 ) ) ;
#33050=VECTOR ( 'NONE', #33128, 1000.000000000000000 ) ;
#33059=DIRECTION ( 'NONE',  ( 0.000000000000000000, 0.000000000000000000, -1.000000000000000000 ) ) ;
#33063=DIRECTION ( 'NONE',  ( 0.000000000000000000, 0.000000000000000000, -1.000000000000000000 ) ) ;
#33069=ORIENTED_EDGE ( 'NONE', *, *, #27524, .T. ) ;
#33082=VERTEX_POINT ( 'NONE', #11924 ) ;
#33128=DIRECTION ( 'NONE',  ( 0.000000000000000000, 0.000000000000000000, 1.000000000000000000 ) ) ;
#33146=CARTESIAN_POINT ( 'NONE',  ( 154.1026953830863420, 103.9380105690400597, -17.65743994998277699 ) ) ;
#33156=DIRECTION ( 'NONE',  ( -0.9770330068457271366, 0.000000000000000000, -0.2130880182788259247 ) ) ;
#33208=ADVANCED_FACE ( 'NONE', ( #45194 ), #49782, .F. ) ;
#33259=AXIS2_PLACEMENT_3D ( 'NONE', #23921, #7783, #12130 ) ;
#33281=VECTOR ( 'NONE', #10287, 1000.000000000000000 ) ;
#33326=EDGE_CURVE ( 'NONE', #23001, #30787, #33696, .T. ) ;
#33351=VERTEX_POINT ( 'NONE', #26748 ) ;
#33361=EDGE_CURVE ( 'NONE', #28480, #4867, #18773, .T. ) ;
#33386=EDGE_CURVE ( 'NONE', #39650, #21642, #34719, .T. ) ;
#33468=ORIENTED_EDGE ( 'NONE', *, *, #27060, .T. ) ;
#33547=EDGE_CURVE ( 'NONE', #30823, #4890, #15273, .T. ) ;
#33550=EDGE_CURVE ( 'NONE', #47536, #25574, #50358, .T. ) ;
#33592=ORIENTED_EDGE ( 'NONE', *, *, #17825, .F. ) ;
#33594=CARTESIAN_POINT ( 'NONE',  ( -5.647304616913629616, 2.688010569040066411, 742.8425600500171413 ) ) ;
#33605=VECTOR ( 'NONE', #37636, 1000.000000000000000 ) ;
#33689=ORIENTED_EDGE ( 'NONE', *, *, #7407, .F. ) ;
#33696=LINE ( 'NONE', #38056, #32729 ) ;
#33729=EDGE_CURVE ( 'NONE', #20088, #17600, #4470, .T. ) ;
#33782=ORIENTED_EDGE ( 'NONE', *, *, #38811, .T. ) ;
#33822=ORIENTED_EDGE ( 'NONE', *, *, #38193, .T. ) ;
#33934=DIRECTION ( 'NONE',  ( 0.000000000000000000, -1.000000000000000000, 0.000000000000000000 ) ) ;
#33971=ORIENTED_EDGE ( 'NONE', *, *, #23017, .T. ) ;
#34012=LINE ( 'NONE', #34261, #22213 ) ;
#34043=ORIENTED_EDGE ( 'NONE', *, *, #4704, .F. ) ;
#34092=EDGE_LOOP ( 'NONE', ( #16596, #7419, #4506, #2211 ) ) ;
#34186=VERTEX_POINT ( 'NONE', #4413 ) ;
#34207=CARTESIAN_POINT ( 'NONE',  ( 154.1026953830863420, 103.9380105690400597, -17.65743994998277699 ) ) ;
#34229=EDGE_LOOP ( 'NONE', ( #44412, #42235, #16928, #47293 ) ) ;
#34260=CARTESIAN_POINT ( 'NONE',  ( 154.1026953830863420, 103.9380105690400597, 22.84256005001721945 ) ) ;
#34261=CARTESIAN_POINT ( 'NONE',  ( -556.8973046169135159, -62.56198943095993315, -64.63743994998280584 ) ) ;
#34277=CARTESIAN_POINT ( 'NONE',  ( 153.2026953830863647, 103.1142457376053727, -17.29493270523947501 ) ) ;
#34310=EDGE_CURVE ( 'NONE', #39650, #31856, #20809, .T. ) ;
#34336=VECTOR ( 'NONE', #19736, 1000.000000000000000 ) ;
#34514=CARTESIAN_POINT ( 'NONE',  ( -5.647304616913629616, -290.4457172416107937, 144.9816133044550668 ) ) ;
#34579=ORIENTED_EDGE ( 'NONE', *, *, #33729, .F. ) ;
#34719=LINE ( 'NONE', #30345, #10590 ) ;
#34726=VECTOR ( 'NONE', #17061, 1000.000000000000000 ) ;
#34785=ORIENTED_EDGE ( 'NONE', *, *, #14919, .F. ) ;
#34858=PLANE ( 'NONE',  #12345 ) ;
#34882=FACE_OUTER_BOUND ( 'NONE', #17925, .T. ) ;
#34921=MECHANICAL_DESIGN_GEOMETRIC_PRESENTATION_REPRESENTATION('',(#29957),#7846);
#34925=AXIS2_PLACEMENT_3D ( 'NONE', #21351, #2117, #17763 ) ;
#34938=EDGE_CURVE ( 'NONE', #25767, #13303, #25240, .T. ) ;
#34975=DIRECTION ( 'NONE',  ( 0.000000000000000000, 1.000000000000000000, 0.000000000000000000 ) ) ;
#34999=EDGE_CURVE ( 'NONE', #22621, #30282, #2152, .T. ) ;
#35026=DIRECTION ( 'NONE',  ( 1.000000000000000000, 0.000000000000000000, 0.000000000000000000 ) ) ;
#35052=DIRECTION ( 'NONE',  ( 0.000000000000000000, -0.000000000000000000, -1.000000000000000000 ) ) ;
#35310=ORIENTED_EDGE ( 'NONE', *, *, #44466, .F. ) ;
#35373=CARTESIAN_POINT ( 'NONE',  ( 195.9526953830863079, -153.9383703589661820, 472.5992458228020610 ) ) ;
#35476=ORIENTED_EDGE ( 'NONE', *, *, #44717, .T. ) ;
#35611=ORIENTED_EDGE ( 'NONE', *, *, #36226, .T. ) ;
#35633=LINE ( 'NONE', #24071, #17681 ) ;
#35678=ORIENTED_EDGE ( 'NONE', *, *, #33729, .T. ) ;
#35681=LINE ( 'NONE', #32320, #11268 ) ;
#35702=CARTESIAN_POINT ( 'NONE',  ( -164.4973046169135955, 70.03596893647589638, -93.79675437945476801 ) ) ;
#35792=LINE ( 'NONE', #8319, #42412 ) ;
#35797=EDGE_LOOP ( 'NONE', ( #46368, #23927, #13334, #32622, #19376, #38382, #20157, #7759 ) ) ;
#35868=ORIENTED_EDGE ( 'NONE', *, *, #8953, .F. ) ;
#35899=VECTOR ( 'NONE', #10942, 1000.000000000000000 ) ;
#35903=FACE_OUTER_BOUND ( 'NONE', #12202, .T. ) ;
#35908=ORIENTED_EDGE ( 'NONE', *, *, #3553, .T. ) ;
#36018=EDGE_LOOP ( 'NONE', ( #39191, #30967, #23382, #28042, #49259 ) ) ;
#36023=VERTEX_POINT ( 'NONE', #15084 ) ;
#36134=ORIENTED_EDGE ( 'NONE', *, *, #36211, .T. ) ;
#36151=DIRECTION ( 'NONE',  ( -0.000000000000000000, -0.3790464617558786942, 0.9253776417389547593 ) ) ;
#36180=ORIENTED_EDGE ( 'NONE', *, *, #32748, .T. ) ;
#36211=EDGE_CURVE ( 'NONE', #18575, #19633, #29408, .T. ) ;
#36226=EDGE_CURVE ( 'NONE', #15550, #10514, #9658, .T. ) ;
#36305=ADVANCED_BREP_SHAPE_REPRESENTATION ( '', ( #22574, #45486 ), #12706 ) ;
#36327=DIRECTION ( 'NONE',  ( -1.000000000000000000, 0.000000000000000000, 0.000000000000000000 ) ) ;
#36381=DIRECTION ( 'NONE',  ( 0.000000000000000000, 1.000000000000000000, -1.822804496942679766E-16 ) ) ;
#36444=PLANE ( 'NONE',  #37239 ) ;
#36477=DIRECTION ( 'NONE',  ( -0.000000000000000000, -0.000000000000000000, -1.000000000000000000 ) ) ;
#36565=EDGE_CURVE ( 'NONE', #39650, #30823, #23100, .T. ) ;
#36593=EDGE_CURVE ( 'NONE', #11397, #32226, #18989, .T. ) ;
#36673=DIRECTION ( 'NONE',  ( 0.000000000000000000, 0.4027858274925602000, 0.9152942571496522906 ) ) ;
#36755=ORIENTED_EDGE ( 'NONE', *, *, #28503, .F. ) ;
#36762=DIRECTION ( 'NONE',  ( -1.000000000000000000, 0.000000000000000000, -0.000000000000000000 ) ) ;
#36792=CARTESIAN_POINT ( 'NONE',  ( -165.3973046169136012, -62.56198943095993315, -94.69675437945474528 ) ) ;
#36827=ORIENTED_EDGE ( 'NONE', *, *, #3553, .F. ) ;
#36896=PLANE ( 'NONE',  #5272 ) ;
#36932=LINE ( 'NONE', #9439, #23248 ) ;
#36959=FACE_OUTER_BOUND ( 'NONE', #37986, .T. ) ;
#36960=DIRECTION ( 'NONE',  ( -1.000000000000000000, 0.000000000000000000, 0.000000000000000000 ) ) ;
#36963=VECTOR ( 'NONE', #8154, 1000.000000000000227 ) ;
#36999=CARTESIAN_POINT ( 'NONE',  ( 154.1026953830863420, 70.03596893647589638, -94.69675437945477370 ) ) ;
#37016=DIRECTION ( 'NONE',  ( 0.2130880182788259525, 0.000000000000000000, -0.9770330068457272477 ) ) ;
#37081=LINE ( 'NONE', #23433, #7909 ) ;
#37093=AXIS2_PLACEMENT_3D ( 'NONE', #50463, #15370, #31283 ) ;
#37150=LINE ( 'NONE', #975, #12837 ) ;
#37166=APPLICATION_CONTEXT ( 'automotive_design' ) ;
#37239=AXIS2_PLACEMENT_3D ( 'NONE', #21517, #16935, #25134 ) ;
#37247=CARTESIAN_POINT ( 'NONE',  ( -164.4973046169135955, 103.0380105690400683, -17.46817021067766973 ) ) ;
#37260=DIRECTION ( 'NONE',  ( -0.000000000000000000, -1.000000000000000000, -0.000000000000000000 ) ) ;
#37326=CARTESIAN_POINT ( 'NONE',  ( -165.3973046169136012, 54.43801056904003133, -17.65743994998275213 ) ) ;
#37378=DIRECTION ( 'NONE',  ( -0.1191452206184307472, 0.000000000000000000, 0.9928768384869219865 ) ) ;
#37382=DIRECTION ( 'NONE',  ( 0.9928768384869219865, 0.000000000000000000, 0.1191452206184307749 ) ) ;
#37386=DIRECTION ( 'NONE',  ( 0.000000000000000000, 1.000000000000000000, 0.000000000000000000 ) ) ;
#37418=FACE_OUTER_BOUND ( 'NONE', #46796, .T. ) ;
#37473=CARTESIAN_POINT ( 'NONE',  ( 370.7621192902014968, 69.44873401059479079, -93.79675437945473959 ) ) ;
#37509=CARTESIAN_POINT ( 'NONE',  ( 196.8526953830863135, -154.8119894309599260, 472.8425600500171981 ) ) ;
#37561=DIRECTION ( 'NONE',  ( 0.000000000000000000, -1.000000000000000000, -0.000000000000000000 ) ) ;
#37620=EDGE_CURVE ( 'NONE', #25767, #15550, #50210, .T. ) ;
#37636=DIRECTION ( 'NONE',  ( -0.000000000000000000, 0.000000000000000000, 1.000000000000000000 ) ) ;
#37669=DIRECTION ( 'NONE',  ( 0.2130880182788259525, 0.000000000000000000, -0.9770330068457272477 ) ) ;
#37758=PLANE ( 'NONE',  #8510 ) ;
#37804=VECTOR ( 'NONE', #20179, 1000.000000000000114 ) ;
#37807=CARTESIAN_POINT ( 'NONE',  ( -165.3973046169136012, -62.56198943095993315, -17.65743994998275213 ) ) ;
#37872=LINE ( 'NONE', #29391, #28773 ) ;
#37986=EDGE_LOOP ( 'NONE', ( #33468, #35476, #31396, #4096 ) ) ;
#38007=DIRECTION ( 'NONE',  ( 0.000000000000000000, 0.000000000000000000, -1.000000000000000000 ) ) ;
#38056=CARTESIAN_POINT ( 'NONE',  ( 154.1026953830863420, -98.56198943095992604, -17.65743994998277699 ) ) ;
#38077=ORIENTED_EDGE ( 'NONE', *, *, #9520, .T. ) ;
#38110=ADVANCED_FACE ( 'NONE', ( #15268 ), #3706, .F. ) ;
#38193=EDGE_CURVE ( 'NONE', #15132, #26345, #44702, .T. ) ;
#38201=ORIENTED_EDGE ( 'NONE', *, *, #4264, .F. ) ;
#38247=ORIENTED_EDGE ( 'NONE', *, *, #32563, .T. ) ;
#38260=ORIENTED_EDGE ( 'NONE', *, *, #41993, .F. ) ;
#38315=CARTESIAN_POINT ( 'NONE',  ( -208.1473046169136580, -154.8119894309599260, 22.84256005001721945 ) ) ;
#38317=ADVANCED_FACE ( 'NONE', ( #10831 ), #14681, .T. ) ;
#38336=LINE ( 'NONE', #26270, #1347 ) ;
#38354=ORIENTED_EDGE ( 'NONE', *, *, #44717, .F. ) ;
#38382=ORIENTED_EDGE ( 'NONE', *, *, #22038, .T. ) ;
#38391=ORIENTED_EDGE ( 'NONE', *, *, #40873, .F. ) ;
#38528=VERTEX_POINT ( 'NONE', #29018 ) ;
#38536=DIRECTION ( 'NONE',  ( -1.000000000000000000, 0.000000000000000000, 0.000000000000000000 ) ) ;
#38592=CARTESIAN_POINT ( 'NONE',  ( -50.13037131770489907, -41.71198943095993172, 741.9425600500172777 ) ) ;
#38707=CARTESIAN_POINT ( 'NONE',  ( 154.1026953830863420, -98.56198943095992604, -17.65743994998277699 ) ) ;
#38729=VECTOR ( 'NONE', #987, 1000.000000000000000 ) ;
#38770=VERTEX_POINT ( 'NONE', #43588 ) ;
#38775=EDGE_CURVE ( 'NONE', #38770, #12440, #43839, .T. ) ;
#38784=ORIENTED_EDGE ( 'NONE', *, *, #12729, .T. ) ;
#38811=EDGE_CURVE ( 'NONE', #12974, #10514, #29708, .T. ) ;
#38827=CARTESIAN_POINT ( 'NONE',  ( -165.3973046169136012, -62.56198943095993315, -17.65743994998275213 ) ) ;
#38872=CARTESIAN_POINT ( 'NONE',  ( 153.2026953830863647, -97.66198943095992036, -17.65743994998277699 ) ) ;
#38892=CARTESIAN_POINT ( 'NONE',  ( -208.1473046169136580, 160.1880105690400171, 472.8425600500171981 ) ) ;
#38949=PLANE ( 'NONE',  #19915 ) ;
#38955=ORIENTED_EDGE ( 'NONE', *, *, #31003, .T. ) ;
#39012=DIRECTION ( 'NONE',  ( 0.000000000000000000, -1.822804496942679766E-16, -1.000000000000000000 ) ) ;
#39029=VECTOR ( 'NONE', #1712, 1000.000000000000000 ) ;
#39191=ORIENTED_EDGE ( 'NONE', *, *, #45223, .F. ) ;
#39289=PLANE ( 'NONE',  #40336 ) ;
#39306=ORIENTED_EDGE ( 'NONE', *, *, #43053, .T. ) ;
#39359=ORIENTED_EDGE ( 'NONE', *, *, #45308, .T. ) ;
#39369=AXIS2_PLACEMENT_3D ( 'NONE', #25055, #40952, #37382 ) ;
#39420=EDGE_CURVE ( 'NONE', #4890, #30787, #17729, .T. ) ;
#39474=LINE ( 'NONE', #40474, #12726 ) ;
#39530=LINE ( 'NONE', #43603, #19991 ) ;
#39612=ORIENTED_EDGE ( 'NONE', *, *, #1719, .T. ) ;
#39650=VERTEX_POINT ( 'NONE', #47162 ) ;
#39740=AXIS2_PLACEMENT_3D ( 'NONE', #29828, #10072, #41375 ) ;
#39760=VECTOR ( 'NONE', #8177, 1000.000000000000000 ) ;
#39789=VECTOR ( 'NONE', #41935, 1000.000000000000000 ) ;
#39863=DIRECTION ( 'NONE',  ( -0.8637789008984334549, 0.000000000000000000, 0.5038710255240862468 ) ) ;
#39868=VECTOR ( 'NONE', #28444, 1000.000000000000000 ) ;
#39999=CARTESIAN_POINT ( 'NONE',  ( -556.8973046169135159, 53.53801056904005407, -64.63743994998280584 ) ) ;
#40003=ADVANCED_FACE ( 'NONE', ( #12483 ), #8149, .T. ) ;
#40009=DIRECTION ( 'NONE',  ( 0.000000000000000000, -1.000000000000000000, 0.000000000000000000 ) ) ;
#40046=ORIENTED_EDGE ( 'NONE', *, *, #4832, .T. ) ;
#40050=CARTESIAN_POINT ( 'NONE',  ( -207.2473046169136808, -154.8119894309599260, 472.8425600500171981 ) ) ;
#40059=FACE_OUTER_BOUND ( 'NONE', #48122, .T. ) ;
#40122=LINE ( 'NONE', #32937, #17941 ) ;
#40151=ORIENTED_EDGE ( 'NONE', *, *, #34310, .T. ) ;
#40156=EDGE_LOOP ( 'NONE', ( #18588, #7656, #43244, #27276 ) ) ;
#40281=VERTEX_POINT ( 'NONE', #25199 ) ;
#40304=PLANE ( 'NONE',  #27787 ) ;
#40336=AXIS2_PLACEMENT_3D ( 'NONE', #40050, #4873, #43620 ) ;
#40348=ORIENTED_EDGE ( 'NONE', *, *, #2519, .T. ) ;
#40422=EDGE_LOOP ( 'NONE', ( #38260, #17784, #3938, #40151 ) ) ;
#40474=CARTESIAN_POINT ( 'NONE',  ( -50.64730461691362962, -42.31198943095992604, 742.8425600500171413 ) ) ;
#40677=LINE ( 'NONE', #1429, #34726 ) ;
#40709=EDGE_LOOP ( 'NONE', ( #40348, #10370, #14880, #49203 ) ) ;
#40789=CARTESIAN_POINT ( 'NONE',  ( 195.9526953830863079, -154.8119894309599260, 472.8425600500171981 ) ) ;
#40810=DIRECTION ( 'NONE',  ( 0.000000000000000000, -1.000000000000000000, 0.000000000000000000 ) ) ;
#40813=EDGE_CURVE ( 'NONE', #30497, #44652, #3541, .T. ) ;
#40850=ORIENTED_EDGE ( 'NONE', *, *, #7407, .T. ) ;
#40852=FACE_OUTER_BOUND ( 'NONE', #31619, .T. ) ;
#40873=EDGE_CURVE ( 'NONE', #20963, #29505, #46616, .T. ) ;
#40890=VECTOR ( 'NONE', #8566, 1000.000000000000000 ) ;
#40925=LINE ( 'NONE', #32993, #20104 ) ;
#40935=AXIS2_PLACEMENT_3D ( 'NONE', #10271, #45129, #5653 ) ;
#40952=DIRECTION ( 'NONE',  ( -0.1191452206184307888, 0.000000000000000000, 0.9928768384869220975 ) ) ;
#40972=DIRECTION ( 'NONE',  ( 0.000000000000000000, 0.000000000000000000, -1.000000000000000000 ) ) ;
#40978=LINE ( 'NONE', #8916, #43369 ) ;
#40989=CARTESIAN_POINT ( 'NONE',  ( -164.4973046169135955, -97.66198943095992036, -17.48025818148969890 ) ) ;
#41066=AXIS2_PLACEMENT_3D ( 'NONE', #31028, #14598, #10747 ) ;
#41087=PLANE ( 'NONE',  #30417 ) ;
#41146=DIRECTION ( 'NONE',  ( -0.4740998230350174647, -0.3386427307392981256, -0.8127425537743155903 ) ) ;
#41203=DIRECTION ( 'NONE',  ( 0.000000000000000000, 0.4027858274925602000, 0.9152942571496522906 ) ) ;
#41226=ORIENTED_EDGE ( 'NONE', *, *, #15392, .F. ) ;
#41314=AXIS2_PLACEMENT_3D ( 'NONE', #47159, #39012, #15397 ) ;
#41345=AXIS2_PLACEMENT_3D ( 'NONE', #33594, #16491, #49183 ) ;
#41375=DIRECTION ( 'NONE',  ( 0.5038710255240859137, 0.000000000000000000, -0.8637789008984335659 ) ) ;
#41415=VECTOR ( 'NONE', #28060, 1000.000000000000000 ) ;
#41445=CARTESIAN_POINT ( 'NONE',  ( -556.8973046169135159, 54.43801056904003133, -64.63743994998280584 ) ) ;
#41472=VERTEX_POINT ( 'NONE', #17817 ) ;
#41530=VERTEX_POINT ( 'NONE', #27564 ) ;
#41677=ORIENTED_EDGE ( 'NONE', *, *, #33361, .T. ) ;
#41766=ORIENTED_EDGE ( 'NONE', *, *, #22110, .T. ) ;
#41860=ADVANCED_FACE ( 'NONE', ( #35903, #42805 ), #11272, .F. ) ;
#41910=DIRECTION ( 'NONE',  ( -1.000000000000000000, 0.000000000000000000, 0.000000000000000000 ) ) ;
#41935=DIRECTION ( 'NONE',  ( -0.000000000000000000, -1.000000000000000000, -0.000000000000000000 ) ) ;
#41993=EDGE_CURVE ( 'NONE', #33082, #31856, #12522, .T. ) ;
#42056=EDGE_LOOP ( 'NONE', ( #28754, #33822, #14641, #23635 ) ) ;
#42165=ORIENTED_EDGE ( 'NONE', *, *, #40813, .F. ) ;
#42179=LINE ( 'NONE', #7047, #8121 ) ;
#42219=DIRECTION ( 'NONE',  ( -0.000000000000000000, -0.000000000000000000, 1.000000000000000000 ) ) ;
#42235=ORIENTED_EDGE ( 'NONE', *, *, #28799, .F. ) ;
#42266=EDGE_CURVE ( 'NONE', #7200, #357, #16075, .T. ) ;
#42267=LINE ( 'NONE', #3005, #29494 ) ;
#42412=VECTOR ( 'NONE', #24219, 1000.000000000000114 ) ;
#42525=EDGE_CURVE ( 'NONE', #36023, #30497, #30922, .T. ) ;
#42690=DIRECTION ( 'NONE',  ( 0.000000000000000000, -0.3846153846153845812, -0.9230769230769231282 ) ) ;
#42730=VERTEX_POINT ( 'NONE', #4959 ) ;
#42764=VECTOR ( 'NONE', #25226, 1000.000000000000227 ) ;
#42805=FACE_BOUND ( 'NONE', #5892, .T. ) ;
#42832=VERTEX_POINT ( 'NONE', #45693 ) ;
#42901=PLANE ( 'NONE',  #33259 ) ;
#43036=LINE ( 'NONE', #14837, #6228 ) ;
#43053=EDGE_CURVE ( 'NONE', #22708, #28480, #4150, .T. ) ;
#43064=CARTESIAN_POINT ( 'NONE',  ( -165.3973046169136012, -98.56198943095992604, -17.65743994998275213 ) ) ;
#43124=CARTESIAN_POINT ( 'NONE',  ( 196.8526953830863135, -154.8119894309599260, 22.84256005001721945 ) ) ;
#43139=LINE ( 'NONE', #46693, #43858 ) ;
#43201=PLANE ( 'NONE',  #5540 ) ;
#43244=ORIENTED_EDGE ( 'NONE', *, *, #34310, .F. ) ;
#43314=DIRECTION ( 'NONE',  ( 0.000000000000000000, 1.000000000000000000, 0.000000000000000000 ) ) ;
#43369=VECTOR ( 'NONE', #13762, 1000.000000000000000 ) ;
#43549=EDGE_CURVE ( 'NONE', #15492, #46409, #30379, .T. ) ;
#43577=CARTESIAN_POINT ( 'NONE',  ( 195.9526953830863079, -154.8119894309599260, 470.5025600500171095 ) ) ;
#43588=CARTESIAN_POINT ( 'NONE',  ( 195.9526953830863079, 159.2880105690400399, 472.5992458228020610 ) ) ;
#43592=FACE_OUTER_BOUND ( 'NONE', #29869, .T. ) ;
#43603=CARTESIAN_POINT ( 'NONE',  ( -208.1473046169136580, 160.1880105690400171, 22.84256005001721945 ) ) ;
#43605=LINE ( 'NONE', #47928, #43974 ) ;
#43620=DIRECTION ( 'NONE',  ( 0.000000000000000000, 0.000000000000000000, -1.000000000000000000 ) ) ;
#43648=CARTESIAN_POINT ( 'NONE',  ( -164.4973046169135387, 103.0380105690400683, -17.65743994998277699 ) ) ;
#43651=CARTESIAN_POINT ( 'NONE',  ( -207.2473046169136808, -153.9812202001906769, 472.4964062038633870 ) ) ;
#43672=DIRECTION ( 'NONE',  ( 0.000000000000000000, -0.000000000000000000, 1.000000000000000000 ) ) ;
#43674=ORIENTED_EDGE ( 'NONE', *, *, #40813, .T. ) ;
#43689=ADVANCED_FACE ( 'NONE', ( #8050 ), #31664, .F. ) ;
#43690=CARTESIAN_POINT ( 'NONE',  ( -165.3973046169136012, -98.56198943095992604, -17.65743994998277699 ) ) ;
#43692=DIRECTION ( 'NONE',  ( 1.000000000000000000, -0.000000000000000000, 0.000000000000000000 ) ) ;
#43839=LINE ( 'NONE', #47151, #30514 ) ;
#43843=PLANE ( 'NONE',  #41314 ) ;
#43858=VECTOR ( 'NONE', #15434, 1000.000000000000000 ) ;
#43974=VECTOR ( 'NONE', #36960, 1000.000000000000000 ) ;
#43984=ORIENTED_EDGE ( 'NONE', *, *, #42266, .T. ) ;
#43988=CARTESIAN_POINT ( 'NONE',  ( -165.3973046169136012, 54.43801056904003133, -94.69675437945474528 ) ) ;
#44056=ADVANCED_FACE ( 'NONE', ( #8749 ), #39289, .T. ) ;
#44062=CARTESIAN_POINT ( 'NONE',  ( -556.8973046169135159, 54.43801056904003133, -64.63743994998280584 ) ) ;
#44078=LINE ( 'NONE', #24602, #2078 ) ;
#44105=EDGE_CURVE ( 'NONE', #15550, #42730, #25151, .T. ) ;
#44232=ORIENTED_EDGE ( 'NONE', *, *, #8953, .T. ) ;
#44237=DIRECTION ( 'NONE',  ( 8.357767709911579088E-16, -1.000000000000000000, 1.822804496942680259E-16 ) ) ;
#44246=ORIENTED_EDGE ( 'NONE', *, *, #33547, .F. ) ;
#44321=CARTESIAN_POINT ( 'NONE',  ( 195.9526953830863079, 159.2880105690400399, 472.8425600500171981 ) ) ;
#44345=DIRECTION ( 'NONE',  ( 0.000000000000000000, -1.000000000000000000, 1.822804496942679766E-16 ) ) ;
#44374=ADVANCED_FACE ( 'NONE', ( #34882 ), #8179, .F. ) ;
#44412=ORIENTED_EDGE ( 'NONE', *, *, #13563, .T. ) ;
#44417=CARTESIAN_POINT ( 'NONE',  ( -165.3973046169136012, 54.43801056904003133, -17.65743994998275213 ) ) ;
#44454=EDGE_LOOP ( 'NONE', ( #10441, #41226, #5757, #24139 ) ) ;
#44466=EDGE_CURVE ( 'NONE', #22708, #25574, #1492, .T. ) ;
#44500=ORIENTED_EDGE ( 'NONE', *, *, #9216, .F. ) ;
#44511=VECTOR ( 'NONE', #37260, 1000.000000000000000 ) ;
#44514=FACE_OUTER_BOUND ( 'NONE', #44454, .T. ) ;
#44523=CARTESIAN_POINT ( 'NONE',  ( -165.3973046169136012, 70.03596893647589638, -94.69675437945477370 ) ) ;
#44560=DIRECTION ( 'NONE',  ( 0.000000000000000000, -0.000000000000000000, 1.000000000000000000 ) ) ;
#44562=ORIENTED_EDGE ( 'NONE', *, *, #5165, .T. ) ;
#44597=ORIENTED_EDGE ( 'NONE', *, *, #6729, .F. ) ;
#44606=DIRECTION ( 'NONE',  ( -1.000000000000000000, 0.000000000000000000, 0.000000000000000000 ) ) ;
#44624=EDGE_LOOP ( 'NONE', ( #22272, #17318, #43984, #40046 ) ) ;
#44652=VERTEX_POINT ( 'NONE', #50335 ) ;
#44702=LINE ( 'NONE', #37807, #42764 ) ;
#44717=EDGE_CURVE ( 'NONE', #20659, #22708, #47259, .T. ) ;
#44750=ORIENTED_EDGE ( 'NONE', *, *, #36211, .F. ) ;
#44823=LINE ( 'NONE', #44321, #16000 ) ;
#45006=DIRECTION ( 'NONE',  ( 0.9770330068457271366, 0.000000000000000000, 0.2130880182788258970 ) ) ;
#45094=DIRECTION ( 'NONE',  ( 0.9770330068457271366, -0.000000000000000000, 0.2130880182788259247 ) ) ;
#45129=DIRECTION ( 'NONE',  ( 0.8637789008984335659, -0.000000000000000000, 0.5038710255240859137 ) ) ;
#45187=PLANE ( 'NONE',  #39740 ) ;
#45194=FACE_OUTER_BOUND ( 'NONE', #40156, .T. ) ;
#45223=EDGE_CURVE ( 'NONE', #16952, #22476, #29504, .T. ) ;
#45308=EDGE_CURVE ( 'NONE', #41530, #41472, #23837, .T. ) ;
#45403=CARTESIAN_POINT ( 'NONE',  ( -543.3973046169135159, 54.43801056904003133, -177.1374399499827916 ) ) ;
#45418=VECTOR ( 'NONE', #4325, 1000.000000000000000 ) ;
#45433=( NAMED_UNIT ( * ) PLANE_ANGLE_UNIT ( ) SI_UNIT ( $, .RADIAN. ) );
#45440=FACE_OUTER_BOUND ( 'NONE', #49037, .T. ) ;
#45457=ORIENTED_EDGE ( 'NONE', *, *, #10925, .F. ) ;
#45472=ORIENTED_EDGE ( 'NONE', *, *, #50675, .T. ) ;
#45486=AXIS2_PLACEMENT_3D ( 'NONE', #31923, #7813, #35026 ) ;
#45518=CARTESIAN_POINT ( 'NONE',  ( 39.35269538308637038, -42.31198943095992604, 742.8425600500171413 ) ) ;
#45693=CARTESIAN_POINT ( 'NONE',  ( 196.8526953830863420, 160.1880105690400455, 472.8425600500170844 ) ) ;
#45762=DIRECTION ( 'NONE',  ( 1.000000000000000000, -0.000000000000000000, -0.000000000000000000 ) ) ;
#45765=DIRECTION ( 'NONE',  ( 0.1191452206184307472, 0.000000000000000000, -0.9928768384869219865 ) ) ;
#45793=DIRECTION ( 'NONE',  ( 0.000000000000000000, 0.000000000000000000, -1.000000000000000000 ) ) ;
#45848=ORIENTED_EDGE ( 'NONE', *, *, #16934, .T. ) ;
#45872=ORIENTED_EDGE ( 'NONE', *, *, #4704, .T. ) ;
#45891=ORIENTED_EDGE ( 'NONE', *, *, #10726, .T. ) ;
#46041=DIRECTION ( 'NONE',  ( 1.000000000000000000, 0.000000000000000000, 0.000000000000000000 ) ) ;
#46082=VERTEX_POINT ( 'NONE', #32613 ) ;
#46084=CARTESIAN_POINT ( 'NONE',  ( -5.647304616913629616, -62.56198943095990472, 22.84256005001721945 ) ) ;
#46169=DIRECTION ( 'NONE',  ( 0.000000000000000000, 0.3790464617558786942, -0.9253776417389547593 ) ) ;
#46179=EDGE_CURVE ( 'NONE', #10514, #30357, #20550, .T. ) ;
#46201=DIRECTION ( 'NONE',  ( 1.000000000000000000, 0.000000000000000000, 0.000000000000000000 ) ) ;
#46270=VECTOR ( 'NONE', #24539, 1000.000000000000000 ) ;
#46272=LINE ( 'NONE', #26563, #25046 ) ;
#46321=DIRECTION ( 'NONE',  ( -0.000000000000000000, -1.000000000000000000, -0.000000000000000000 ) ) ;
#46358=PLANE ( 'NONE',  #6308 ) ;
#46368=ORIENTED_EDGE ( 'NONE', *, *, #37620, .T. ) ;
#46409=VERTEX_POINT ( 'NONE', #43577 ) ;
#46464=UNCERTAINTY_MEASURE_WITH_UNIT (LENGTH_MEASURE( 1.000000000000000082E-05 ), #48263, 'distance_accuracy_value', 'NONE');
#46500=PLANE ( 'NONE',  #50366 ) ;
#46523=VECTOR ( 'NONE', #17517, 999.9999999999998863 ) ;
#46578=EDGE_CURVE ( 'NONE', #22476, #14628, #36932, .T. ) ;
#46600=AXIS2_PLACEMENT_3D ( 'NONE', #17181, #10241, #9475 ) ;
#46616=LINE ( 'NONE', #26903, #39760 ) ;
#46629=ADVANCED_FACE ( 'NONE', ( #24848, #14034 ), #13780, .T. ) ;
#46681=ADVANCED_FACE ( 'NONE', ( #3242 ), #49657, .F. ) ;
#46693=CARTESIAN_POINT ( 'NONE',  ( -207.2473046169136808, -154.8119894309599260, 472.5992458228020610 ) ) ;
#46753=FACE_OUTER_BOUND ( 'NONE', #19060, .T. ) ;
#46781=ORIENTED_EDGE ( 'NONE', *, *, #32509, .F. ) ;
#46796=EDGE_LOOP ( 'NONE', ( #45872, #20777, #959, #31732 ) ) ;
#46803=LINE ( 'NONE', #47058, #23793 ) ;
#46831=CARTESIAN_POINT ( 'NONE',  ( -164.4973046169135955, -97.72914955339486198, -17.31629813440246579 ) ) ;
#46871=CARTESIAN_POINT ( 'NONE',  ( 154.1026953830863420, -97.66198943095992036, 23.74256005001722158 ) ) ;
#47025=CARTESIAN_POINT ( 'NONE',  ( -165.3973046169136012, 54.43801056904003133, -94.69675437945474528 ) ) ;
#47058=CARTESIAN_POINT ( 'NONE',  ( -208.1473046169136580, -154.8119894309599260, 470.5025600500171095 ) ) ;
#47068=CARTESIAN_POINT ( 'NONE',  ( -556.8973046169135159, -61.66198943095990614, -64.63743994998280584 ) ) ;
#47151=CARTESIAN_POINT ( 'NONE',  ( 93.25146017538654064, 159.2880105690400399, 648.6585061788589428 ) ) ;
#47159=CARTESIAN_POINT ( 'NONE',  ( 370.7621192902014968, 70.03596893647589638, -94.69675437945477370 ) ) ;
#47162=CARTESIAN_POINT ( 'NONE',  ( -165.3973046169136012, 103.9380105690400597, -17.65743994998277699 ) ) ;
#47225=ORIENTED_EDGE ( 'NONE', *, *, #1804, .T. ) ;
#47253=ORIENTED_EDGE ( 'NONE', *, *, #22038, .F. ) ;
#47259=LINE ( 'NONE', #12896, #27261 ) ;
#47293=ORIENTED_EDGE ( 'NONE', *, *, #9600, .T. ) ;
#47299=EDGE_LOOP ( 'NONE', ( #1071, #31920, #44562, #668 ) ) ;
#47366=ORIENTED_EDGE ( 'NONE', *, *, #44105, .F. ) ;
#47379=DIRECTION ( 'NONE',  ( 1.000000000000000000, 0.000000000000000000, 0.000000000000000000 ) ) ;
#47388=CARTESIAN_POINT ( 'NONE',  ( 153.2026953830863647, -98.56198943095992604, 23.74256005001722158 ) ) ;
#47396=ORIENTED_EDGE ( 'NONE', *, *, #1066, .T. ) ;
#47421=ADVANCED_FACE ( 'NONE', ( #43592 ), #43843, .T. ) ;
#47438=LINE ( 'NONE', #12324, #19685 ) ;
#47455=( NAMED_UNIT ( * ) SI_UNIT ( $, .STERADIAN. ) SOLID_ANGLE_UNIT ( ) );
#47523=DIRECTION ( 'NONE',  ( 0.000000000000000000, 0.000000000000000000, -1.000000000000000000 ) ) ;
#47536=VERTEX_POINT ( 'NONE', #13792 ) ;
#47619=VECTOR ( 'NONE', #36477, 1000.000000000000000 ) ;
#47749=VECTOR ( 'NONE', #37386, 1000.000000000000000 ) ;
#47790=ADVANCED_FACE ( 'NONE', ( #24053 ), #38949, .F. ) ;
#47911=ORIENTED_EDGE ( 'NONE', *, *, #20076, .T. ) ;
#47928=CARTESIAN_POINT ( 'NONE',  ( 370.7621192902014968, -67.00570555996102939, -94.69675437945474528 ) ) ;
#47953=DIRECTION ( 'NONE',  ( -0.1191452206184307888, 0.000000000000000000, 0.9928768384869220975 ) ) ;
#47956=( NAMED_UNIT ( * ) PLANE_ANGLE_UNIT ( ) SI_UNIT ( $, .RADIAN. ) );
#48045=EDGE_CURVE ( 'NONE', #47536, #25227, #3908, .T. ) ;
#48122=EDGE_LOOP ( 'NONE', ( #28592, #11632, #20349, #33971 ) ) ;
#48169=ORIENTED_EDGE ( 'NONE', *, *, #17825, .T. ) ;
#48196=ADVANCED_FACE ( 'NONE', ( #21328 ), #13119, .T. ) ;
#48206=VECTOR ( 'NONE', #40810, 1000.000000000000000 ) ;
#48227=LINE ( 'NONE', #43651, #50668 ) ;
#48231=CARTESIAN_POINT ( 'NONE',  ( -165.4943081650523027, 53.53801056904005407, -93.79675437945476801 ) ) ;
#48238=VECTOR ( 'NONE', #46201, 1000.000000000000000 ) ;
#48242=LINE ( 'NONE', #44417, #49350 ) ;
#48249=DIRECTION ( 'NONE',  ( 1.000000000000000000, -0.000000000000000000, 0.000000000000000000 ) ) ;
#48263=( LENGTH_UNIT ( ) NAMED_UNIT ( * ) SI_UNIT ( .MILLI., .METRE. ) );
#48270=ORIENTED_EDGE ( 'NONE', *, *, #36226, .F. ) ;
#48310=VECTOR ( 'NONE', #12421, 1000.000000000000000 ) ;
#48339=CARTESIAN_POINT ( 'NONE',  ( -164.4973046169135955, -61.66198943095990614, -18.45589678844777382 ) ) ;
#48388=ADVANCED_FACE ( 'NONE', ( #50238 ), #37758, .T. ) ;
#48456=CARTESIAN_POINT ( 'NONE',  ( 298.7932379171858770, 232.7719218785460953, 296.3011729072026128 ) ) ;
#48624=VERTEX_POINT ( 'NONE', #27207 ) ;
#48778=CARTESIAN_POINT ( 'NONE',  ( 195.9526953830863079, 159.2880105690400399, 23.74256005001722158 ) ) ;
#48814=VECTOR ( 'NONE', #18728, 1000.000000000000000 ) ;
#48833=CARTESIAN_POINT ( 'NONE',  ( 153.2026953830863647, -66.40178110878292728, -93.79675437945473959 ) ) ;
#48848=FACE_BOUND ( 'NONE', #12064, .T. ) ;
#49015=ADVANCED_FACE ( 'NONE', ( #5555 ), #36896, .F. ) ;
#49028=DIRECTION ( 'NONE',  ( -0.000000000000000000, -0.000000000000000000, 1.000000000000000000 ) ) ;
#49037=EDGE_LOOP ( 'NONE', ( #32885, #30689, #24686, #2284, #4310 ) ) ;
#49054=EDGE_LOOP ( 'NONE', ( #49190, #1326, #6163, #44246 ) ) ;
#49086=ORIENTED_EDGE ( 'NONE', *, *, #38811, .F. ) ;
#49090=CARTESIAN_POINT ( 'NONE',  ( 154.1026953830863420, 103.9380105690400597, -17.65743994998277699 ) ) ;
#49183=DIRECTION ( 'NONE',  ( -1.000000000000000000, 0.000000000000000000, -0.000000000000000000 ) ) ;
#49190=ORIENTED_EDGE ( 'NONE', *, *, #32827, .F. ) ;
#49203=ORIENTED_EDGE ( 'NONE', *, *, #28799, .T. ) ;
#49259=ORIENTED_EDGE ( 'NONE', *, *, #19335, .T. ) ;
#49338=CARTESIAN_POINT ( 'NONE',  ( 154.1026953830863420, -98.56198943095992604, 22.84256005001721945 ) ) ;
#49350=VECTOR ( 'NONE', #13135, 1000.000000000000000 ) ;
#49381=FACE_OUTER_BOUND ( 'NONE', #10274, .T. ) ;
#49517=ORIENTED_EDGE ( 'NONE', *, *, #39420, .T. ) ;
#49539=PRODUCT_DEFINITION_FORMATION_WITH_SPECIFIED_SOURCE ( 'ANY', '', #14677, .NOT_KNOWN. ) ;
#49598=PLANE ( 'NONE',  #9112 ) ;
#49657=PLANE ( 'NONE',  #2770 ) ;
#49677=CARTESIAN_POINT ( 'NONE',  ( -165.3973046169136012, 54.43801056904003133, -17.65743994998275213 ) ) ;
#49747=ADVANCED_FACE ( 'NONE', ( #2275 ), #16731, .F. ) ;
#49782=PLANE ( 'NONE',  #5681 ) ;
#49810=FACE_OUTER_BOUND ( 'NONE', #40422, .T. ) ;
#50029=DIRECTION ( 'NONE',  ( 0.000000000000000000, 0.4027858274925601445, 0.9152942571496521795 ) ) ;
#50121=ORIENTED_EDGE ( 'NONE', *, *, #36593, .F. ) ;
#50206=LINE ( 'NONE', #26672, #1156 ) ;
#50210=LINE ( 'NONE', #10757, #25689 ) ;
#50211=ORIENTED_EDGE ( 'NONE', *, *, #22389, .T. ) ;
#50219=EDGE_LOOP ( 'NONE', ( #15991, #41766, #1227, #33592, #47396 ) ) ;
#50238=FACE_OUTER_BOUND ( 'NONE', #14977, .T. ) ;
#50335=CARTESIAN_POINT ( 'NONE',  ( -164.4973046169135955, -97.66198943095992036, 23.74256005001722158 ) ) ;
#50336=VERTEX_POINT ( 'NONE', #24993 ) ;
#50358=LINE ( 'NONE', #45518, #31968 ) ;
#50366=AXIS2_PLACEMENT_3D ( 'NONE', #11911, #43692, #11393 ) ;
#50463=CARTESIAN_POINT ( 'NONE',  ( 154.1026953830863420, -98.56198943095992604, -17.65743994998277699 ) ) ;
#50557=CARTESIAN_POINT ( 'NONE',  ( -207.2473046169136808, 2.688010569040066411, 23.74256005001722158 ) ) ;
#50581=EDGE_CURVE ( 'NONE', #19633, #50336, #40925, .T. ) ;
#50668=VECTOR ( 'NONE', #4676, 999.9999999999998863 ) ;
#50675=EDGE_CURVE ( 'NONE', #34186, #28480, #29625, .T. ) ;
#50776=COLOUR_RGB('Off White',0.89,0.88,0.83);
#50777=FILL_AREA_STYLE_COLOUR('',#50776);
#50778=FILL_AREA_STYLE('',(#50777));
#50779=SURFACE_STYLE_FILL_AREA(#50778);
#50780=SURFACE_SIDE_STYLE('',(#50779));
#50781=SURFACE_STYLE_USAGE(.BOTH.,#50780);
#50782=PRESENTATION_STYLE_ASSIGNMENT((#50781));
ENDSEC;
END-ISO-10303-21;
